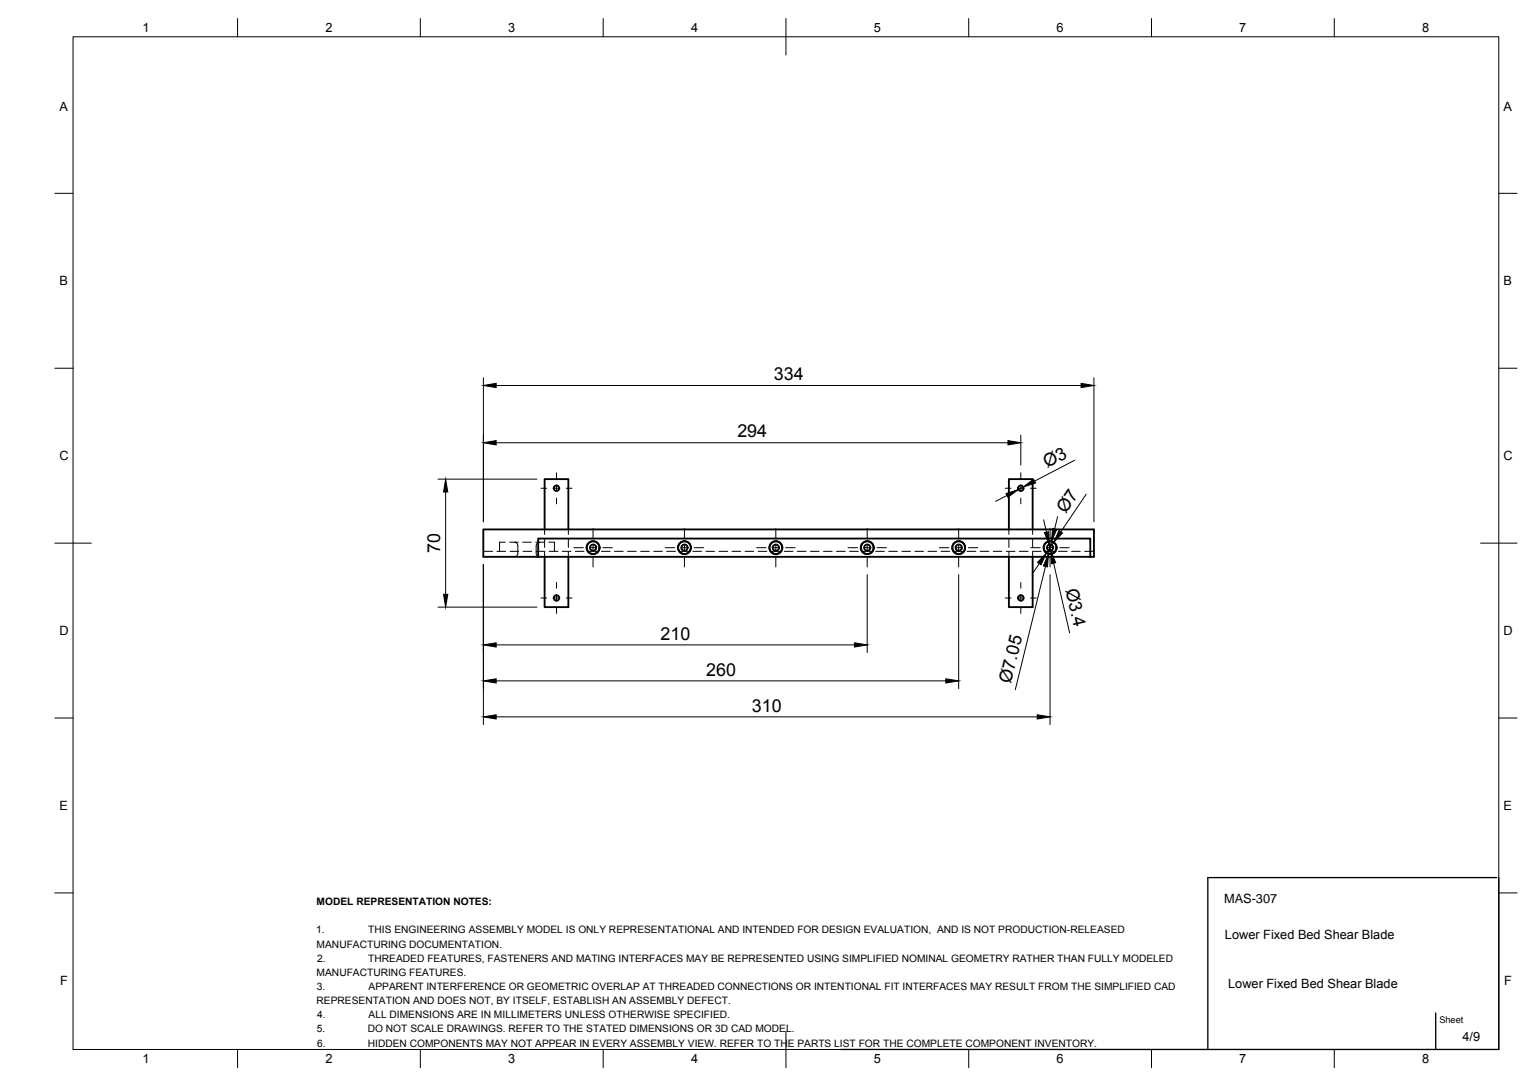
ISO-10303-21;
HEADER;
FILE_DESCRIPTION (('STEP AP214'),
    '1' );
FILE_NAME ('Lower Fixed Bed Shear Blade.step',
    '2026-10-06T07:34:29',
    ( '' ),
    ( '' ),
    'SwSTEP 2.0',
    'SolidWorks 2025',
    '' );
FILE_SCHEMA (( 'AUTOMOTIVE_DESIGN' ));
ENDSEC;

DATA;
#1=ORIENTED_EDGE ( 'NONE', *, *, #36, .T. ) ;
#8=ORIENTED_EDGE ( 'NONE', *, *, #9613, .T. ) ;
#9=EDGE_LOOP ( 'NONE', ( #498, #10940, #14960, #5861, #9835 ) ) ;
#14=LINE ( 'NONE', #12973, #6716 ) ;
#16=VECTOR ( 'NONE', #3003, 1000.000000000000000 ) ;
#17=EDGE_CURVE ( 'NONE', #5528, #10245, #15139, .T. ) ;
#23=DIRECTION ( 'NONE',  ( -0.000000000000000000, 1.156482317317871478E-16, -1.000000000000000000 ) ) ;
#27=ORIENTED_EDGE ( 'NONE', *, *, #13841, .F. ) ;
#29=VECTOR ( 'NONE', #1575, 1000.000000000000000 ) ;
#33=VECTOR ( 'NONE', #1804, 1000.000000000000000 ) ;
#36=EDGE_CURVE ( 'NONE', #15150, #10379, #8408, .T. ) ;
#43=DIRECTION ( 'NONE',  ( 0.000000000000000000, 0.000000000000000000, 1.000000000000000000 ) ) ;
#46=FACE_OUTER_BOUND ( 'NONE', #2849, .T. ) ;
#49=ORIENTED_EDGE ( 'NONE', *, *, #2623, .T. ) ;
#55=CARTESIAN_POINT ( 'NONE',  ( -76.50000000000001421, 19.53993994372674692, -17.50000000000002487 ) ) ;
#59=EDGE_CURVE ( 'NONE', #163, #6601, #13932, .T. ) ;
#61=VERTEX_POINT ( 'NONE', #1883 ) ;
#62=AXIS2_PLACEMENT_3D ( 'NONE', #15140, #11528, #6573 ) ;
#66=ORIENTED_EDGE ( 'NONE', *, *, #14903, .T. ) ;
#80=CIRCLE ( 'NONE', #13699, 3.525000000000000355 ) ;
#81=CARTESIAN_POINT ( 'NONE',  ( -110.0000000000000426, 59.53993994372674337, 10.00000000000000178 ) ) ;
#83=ADVANCED_FACE ( 'NONE', ( #687 ), #5531, .F. ) ;
#86=EDGE_LOOP ( 'NONE', ( #3348, #2604, #2165, #14498 ) ) ;
#93=ORIENTED_EDGE ( 'NONE', *, *, #2529, .F. ) ;
#94=AXIS2_PLACEMENT_3D ( 'NONE', #7418, #12210, #6221 ) ;
#111=ADVANCED_FACE ( 'NONE', ( #1394 ), #10899, .F. ) ;
#114=CARTESIAN_POINT ( 'NONE',  ( -35.99999999999995026, 62.13993994372673768, 18.50000000000140332 ) ) ;
#116=CARTESIAN_POINT ( 'NONE',  ( -108.0000000000000568, 64.53993994372673626, 20.00000000000000355 ) ) ;
#119=CARTESIAN_POINT ( 'NONE',  ( 114.0000000000000568, 64.53993994372673626, 11.50000000000034817 ) ) ;
#126=CARTESIAN_POINT ( 'NONE',  ( 185.1062858801516882, 25.86394065090268057, 18.00000000000000355 ) ) ;
#131=ORIENTED_EDGE ( 'NONE', *, *, #13724, .F. ) ;
#139=CARTESIAN_POINT ( 'NONE',  ( 164.0000000000000568, 64.53993994372673626, 16.70000000000000995 ) ) ;
#147=PLANE ( 'NONE',  #811 ) ;
#162=DIRECTION ( 'NONE',  ( 8.659560562354932858E-17, 0.7071067811865474617, -0.7071067811865474617 ) ) ;
#163=VERTEX_POINT ( 'NONE', #8301 ) ;
#167=ORIENTED_EDGE ( 'NONE', *, *, #13377, .T. ) ;
#178=CARTESIAN_POINT ( 'NONE',  ( -85.99999999999994316, 64.51493994372674479, 18.50000000000175149 ) ) ;
#181=CARTESIAN_POINT ( 'NONE',  ( 200.1062858801516597, 40.86394065090267702, 12.00000000000001066 ) ) ;
#186=DIRECTION ( 'NONE',  ( 0.000000000000000000, 0.000000000000000000, 1.000000000000000000 ) ) ;
#198=DIRECTION ( 'NONE',  ( 0.000000000000000000, 0.000000000000000000, 1.000000000000000000 ) ) ;
#210=EDGE_LOOP ( 'NONE', ( #10445, #12034, #11284, #6545 ) ) ;
#220=DIRECTION ( 'NONE',  ( -0.000000000000000000, 1.486905836551548832E-16, -1.000000000000000000 ) ) ;
#221=ORIENTED_EDGE ( 'NONE', *, *, #12224, .F. ) ;
#222=( GEOMETRIC_REPRESENTATION_CONTEXT ( 3 ) GLOBAL_UNCERTAINTY_ASSIGNED_CONTEXT ( ( #10529 ) ) GLOBAL_UNIT_ASSIGNED_CONTEXT ( ( #15547, #7222, #9271 ) ) REPRESENTATION_CONTEXT ( 'NONE', 'WORKASPACE' ) );
#232=DIRECTION ( 'NONE',  ( -0.000000000000000000, 1.000000000000000000, 1.156482317317871725E-16 ) ) ;
#233=AXIS2_PLACEMENT_3D ( 'NONE', #7331, #6137, #10957 ) ;
#236=LINE ( 'NONE', #6353, #3489 ) ;
#240=DIRECTION ( 'NONE',  ( 0.000000000000000000, -1.000000000000000000, 0.000000000000000000 ) ) ;
#244=EDGE_CURVE ( 'NONE', #1879, #4614, #5269, .T. ) ;
#250=ORIENTED_EDGE ( 'NONE', *, *, #12118, .T. ) ;
#252=CYLINDRICAL_SURFACE ( 'NONE', #13481, 1.700000000000007061 ) ;
#253=EDGE_CURVE ( 'NONE', #2275, #9404, #10915, .T. ) ;
#259=VERTEX_POINT ( 'NONE', #512 ) ;
#262=ADVANCED_FACE ( 'NONE', ( #11203, #355 ), #1639, .F. ) ;
#263=CARTESIAN_POINT ( 'NONE',  ( 14.00000000000004086, 64.53993994372673626, 15.00000000000104983 ) ) ;
#267=DIRECTION ( 'NONE',  ( 0.000000000000000000, -1.000000000000000000, -1.156482317317871478E-16 ) ) ;
#272=CARTESIAN_POINT ( 'NONE',  ( 14.00000000000004086, 62.13993994372673768, 15.00000000000104983 ) ) ;
#275=ORIENTED_EDGE ( 'NONE', *, *, #10508, .T. ) ;
#276=CARTESIAN_POINT ( 'NONE',  ( 215.1062858801516882, 55.86394065090267702, 13.00000000000000178 ) ) ;
#278=EDGE_CURVE ( 'NONE', #319, #8130, #1801, .T. ) ;
#280=DIRECTION ( 'NONE',  ( 0.000000000000000000, 0.000000000000000000, 1.000000000000000000 ) ) ;
#293=ORIENTED_EDGE ( 'NONE', *, *, #8057, .F. ) ;
#299=VERTEX_POINT ( 'NONE', #8683 ) ;
#300=DIRECTION ( 'NONE',  ( 0.000000000000000000, 1.000000000000000000, 0.000000000000000000 ) ) ;
#303=ORIENTED_EDGE ( 'NONE', *, *, #14000, .F. ) ;
#308=CARTESIAN_POINT ( 'NONE',  ( 177.5000000000000853, 17.53993994372673271, 52.49999999999997868 ) ) ;
#309=EDGE_LOOP ( 'NONE', ( #6645, #5526, #11534, #9026 ) ) ;
#312=COLOUR_RGB ( '', 0.08235294, 0.09019608, 0.10196078) ;
#315=ORIENTED_EDGE ( 'NONE', *, *, #1829, .T. ) ;
#319=VERTEX_POINT ( 'NONE', #10023 ) ;
#321=FACE_BOUND ( 'NONE', #9577, .T. ) ;
#324=FACE_OUTER_BOUND ( 'NONE', #11938, .T. ) ;
#327=DIRECTION ( 'NONE',  ( -0.000000000000000000, 1.000000000000000000, 0.000000000000000000 ) ) ;
#337=ORIENTED_EDGE ( 'NONE', *, *, #9909, .T. ) ;
#340=DIRECTION ( 'NONE',  ( -0.000000000000000000, 1.000000000000000000, -0.000000000000000000 ) ) ;
#346=EDGE_CURVE ( 'NONE', #13457, #11923, #1210, .T. ) ;
#348=DIRECTION ( 'NONE',  ( 0.000000000000000000, 0.000000000000000000, 1.000000000000000000 ) ) ;
#349=ORIENTED_EDGE ( 'NONE', *, *, #4874, .F. ) ;
#350=CARTESIAN_POINT ( 'NONE',  ( -70.00000000000000000, 19.53993994372674337, -12.49999999999999467 ) ) ;
#353=FACE_OUTER_BOUND ( 'NONE', #13566, .T. ) ;
#355=FACE_OUTER_BOUND ( 'NONE', #6775, .T. ) ;
#356=LINE ( 'NONE', #15042, #7156 ) ;
#357=CYLINDRICAL_SURFACE ( 'NONE', #6736, 1.700000000000001954 ) ;
#363=FACE_OUTER_BOUND ( 'NONE', #2322, .T. ) ;
#368=EDGE_LOOP ( 'NONE', ( #10873, #2288 ) ) ;
#370=ORIENTED_EDGE ( 'NONE', *, *, #1545, .F. ) ;
#382=EDGE_LOOP ( 'NONE', ( #11195, #13930, #5127, #3542 ) ) ;
#391=CARTESIAN_POINT ( 'NONE',  ( -85.99999999999994316, 62.13993994372673768, 13.30000000000175575 ) ) ;
#402=DIRECTION ( 'NONE',  ( -0.000000000000000000, 1.000000000000000000, -0.000000000000000000 ) ) ;
#404=FACE_BOUND ( 'NONE', #3437, .T. ) ;
#411=VERTEX_POINT ( 'NONE', #1368 ) ;
#413=CARTESIAN_POINT ( 'NONE',  ( -63.50000000000002842, 19.53993994372674337, 9.999999999999998224 ) ) ;
#422=EDGE_CURVE ( 'NONE', #8299, #5528, #13370, .T. ) ;
#428=ORIENTED_EDGE ( 'NONE', *, *, #9080, .F. ) ;
#432=CARTESIAN_POINT ( 'NONE',  ( -70.00000000000000000, 17.53993994372673271, 45.99999999999998579 ) ) ;
#435=VERTEX_POINT ( 'NONE', #5016 ) ;
#438=PRODUCT_DEFINITION_CONTEXT ( 'detailed design', #1607, 'design' ) ;
#449=CARTESIAN_POINT ( 'NONE',  ( 184.0000000000000568, 19.53993994372674337, -10.99999999999999822 ) ) ;
#464=AXIS2_PLACEMENT_3D ( 'NONE', #11793, #3266, #8332 ) ;
#467=EDGE_LOOP ( 'NONE', ( #5925, #93, #1050, #7042 ) ) ;
#469=LINE ( 'NONE', #13437, #12129 ) ;
#470=VERTEX_POINT ( 'NONE', #2334 ) ;
#473=CIRCLE ( 'NONE', #10842, 3.525000000000000355 ) ;
#487=ORIENTED_EDGE ( 'NONE', *, *, #5572, .T. ) ;
#490=ORIENTED_EDGE ( 'NONE', *, *, #10011, .F. ) ;
#497=CARTESIAN_POINT ( 'NONE',  ( -35.99999999999995026, 59.53993994372674337, 13.30000000000139870 ) ) ;
#498=ORIENTED_EDGE ( 'NONE', *, *, #7139, .T. ) ;
#499=FACE_OUTER_BOUND ( 'NONE', #8321, .T. ) ;
#504=ORIENTED_EDGE ( 'NONE', *, *, #12136, .F. ) ;
#512=CARTESIAN_POINT ( 'NONE',  ( 194.0000000000000568, 64.53993994372673626, 10.00000000000000178 ) ) ;
#521=AXIS2_PLACEMENT_3D ( 'NONE', #14117, #9393, #14192 ) ;
#527=ORIENTED_EDGE ( 'NONE', *, *, #1736, .T. ) ;
#546=ORIENTED_EDGE ( 'NONE', *, *, #11091, .T. ) ;
#560=DIRECTION ( 'NONE',  ( -0.000000000000000000, 1.000000000000000000, -0.000000000000000000 ) ) ;
#576=VECTOR ( 'NONE', #13961, 1000.000000000000000 ) ;
#591=VERTEX_POINT ( 'NONE', #3904 ) ;
#596=ADVANCED_FACE ( 'NONE', ( #3241, #7547, #404, #10066, #5321, #12343, #1529 ), #6365, .T. ) ;
#597=VECTOR ( 'NONE', #13500, 1000.000000000000000 ) ;
#598=CARTESIAN_POINT ( 'NONE',  ( 14.00000000000004086, 64.51493994372674479, 11.50000000000105160 ) ) ;
#605=FACE_OUTER_BOUND ( 'NONE', #8179, .T. ) ;
#608=CARTESIAN_POINT ( 'NONE',  ( 200.1062858801516597, 40.86394065090267702, 12.00000000000001066 ) ) ;
#613=CARTESIAN_POINT ( 'NONE',  ( 114.0000000000000568, 59.53993994372674337, 15.00000000000035172 ) ) ;
#614=CARTESIAN_POINT ( 'NONE',  ( 185.1062858801516882, 55.86394065090267702, 18.00000000000000355 ) ) ;
#625=EDGE_CURVE ( 'NONE', #15030, #13622, #4821, .T. ) ;
#627=VERTEX_POINT ( 'NONE', #2292 ) ;
#629=VECTOR ( 'NONE', #6503, 1000.000000000000114 ) ;
#634=VECTOR ( 'NONE', #8882, 1000.000000000000000 ) ;
#641=DIRECTION ( 'NONE',  ( 0.000000000000000000, 0.000000000000000000, 1.000000000000000000 ) ) ;
#644=DIRECTION ( 'NONE',  ( 0.000000000000000000, -1.000000000000000000, 0.000000000000000000 ) ) ;
#646=CARTESIAN_POINT ( 'NONE',  ( 114.0000000000000568, 59.53993994372674337, 13.30000000000035776 ) ) ;
#649=VERTEX_POINT ( 'NONE', #14359 ) ;
#659=EDGE_LOOP ( 'NONE', ( #14595, #131 ) ) ;
#662=FACE_OUTER_BOUND ( 'NONE', #4108, .T. ) ;
#665=DIRECTION ( 'NONE',  ( 0.000000000000000000, 0.000000000000000000, 1.000000000000000000 ) ) ;
#666=ORIENTED_EDGE ( 'NONE', *, *, #11149, .F. ) ;
#668=DIRECTION ( 'NONE',  ( 0.000000000000000000, 0.000000000000000000, -1.000000000000000000 ) ) ;
#669=DIRECTION ( 'NONE',  ( -0.000000000000000000, 1.000000000000000000, -0.000000000000000000 ) ) ;
#670=CARTESIAN_POINT ( 'NONE',  ( 164.0000000000000568, 62.13993994372673768, 15.00000000000000355 ) ) ;
#677=FACE_OUTER_BOUND ( 'NONE', #3082, .T. ) ;
#687=FACE_OUTER_BOUND ( 'NONE', #13168, .T. ) ;
#692=VECTOR ( 'NONE', #1638, 1000.000000000000000 ) ;
#694=ORIENTED_EDGE ( 'NONE', *, *, #8736, .F. ) ;
#701=VERTEX_POINT ( 'NONE', #11853 ) ;
#702=ORIENTED_EDGE ( 'NONE', *, *, #1006, .F. ) ;
#711=DIRECTION ( 'NONE',  ( 1.000000000000000000, 0.000000000000000000, 0.000000000000000000 ) ) ;
#712=DIRECTION ( 'NONE',  ( 1.000000000000000000, 0.000000000000000000, -0.000000000000000000 ) ) ;
#716=CARTESIAN_POINT ( 'NONE',  ( -70.00000000000000000, 17.53993994372673271, 47.49999999999997868 ) ) ;
#728=AXIS2_PLACEMENT_3D ( 'NONE', #4128, #8966, #3036 ) ;
#733=DIRECTION ( 'NONE',  ( 0.000000000000000000, 0.000000000000000000, 1.000000000000000000 ) ) ;
#737=AXIS2_PLACEMENT_3D ( 'NONE', #10217, #240, #15526 ) ;
#741=CYLINDRICAL_SURFACE ( 'NONE', #7444, 3.500000000000001332 ) ;
#747=EDGE_CURVE ( 'NONE', #6193, #15197, #6107, .T. ) ;
#755=CARTESIAN_POINT ( 'NONE',  ( 64.00000000000005684, 64.53993994372673626, 15.00000000000070166 ) ) ;
#759=CARTESIAN_POINT ( 'NONE',  ( 184.0000000000000568, 17.53993994372673271, 47.49999999999997868 ) ) ;
#774=CARTESIAN_POINT ( 'NONE',  ( 64.00000000000005684, 64.53993994372673626, 11.47500000000070131 ) ) ;
#778=ORIENTED_EDGE ( 'NONE', *, *, #7223, .T. ) ;
#782=ORIENTED_EDGE ( 'NONE', *, *, #1484, .F. ) ;
#786=DIRECTION ( 'NONE',  ( 0.000000000000000000, 0.000000000000000000, 1.000000000000000000 ) ) ;
#792=DIRECTION ( 'NONE',  ( 0.000000000000000000, -1.486905836551548832E-16, 1.000000000000000000 ) ) ;
#794=CARTESIAN_POINT ( 'NONE',  ( 14.00000000000004086, 59.53993994372674337, 15.00000000000104983 ) ) ;
#807=ORIENTED_EDGE ( 'NONE', *, *, #7985, .T. ) ;
#811=AXIS2_PLACEMENT_3D ( 'NONE', #8478, #2543, #7216 ) ;
#819=CARTESIAN_POINT ( 'NONE',  ( 200.1062858801516597, 40.86394065090267702, 12.00000000000001066 ) ) ;
#820=ADVANCED_FACE ( 'NONE', ( #7360 ), #12154, .F. ) ;
#821=AXIS2_PLACEMENT_3D ( 'NONE', #7186, #2427, #43 ) ;
#841=DIRECTION ( 'NONE',  ( 0.000000000000000000, -1.000000000000000000, 0.000000000000000000 ) ) ;
#842=CIRCLE ( 'NONE', #12444, 1.499999999999997780 ) ;
#843=DIRECTION ( 'NONE',  ( 0.000000000000000000, 0.000000000000000000, -1.000000000000000000 ) ) ;
#848=ORIENTED_EDGE ( 'NONE', *, *, #6781, .T. ) ;
#851=CIRCLE ( 'NONE', #6656, 1.499999999999997780 ) ;
#855=EDGE_CURVE ( 'NONE', #8929, #14758, #8389, .T. ) ;
#856=EDGE_CURVE ( 'NONE', #10437, #9262, #1951, .T. ) ;
#864=ORIENTED_EDGE ( 'NONE', *, *, #15101, .T. ) ;
#865=CYLINDRICAL_SURFACE ( 'NONE', #11752, 1.699999999999994849 ) ;
#868=VERTEX_POINT ( 'NONE', #5283 ) ;
#871=CARTESIAN_POINT ( 'NONE',  ( 200.1062858801516597, 40.86394065090267702, 16.00000000000001421 ) ) ;
#889=EDGE_CURVE ( 'NONE', #9525, #12618, #11656, .T. ) ;
#891=DIRECTION ( 'NONE',  ( 0.000000000000000000, 1.000000000000000000, 1.156482317317871725E-16 ) ) ;
#899=VERTEX_POINT ( 'NONE', #14266 ) ;
#903=DIRECTION ( 'NONE',  ( 0.000000000000000000, 0.000000000000000000, 1.000000000000000000 ) ) ;
#910=CARTESIAN_POINT ( 'NONE',  ( 64.00000000000005684, 62.13993994372673768, 15.00000000000070166 ) ) ;
#912=CARTESIAN_POINT ( 'NONE',  ( -35.99999999999995026, 62.13993994372673768, 15.00000000000139977 ) ) ;
#917=EDGE_CURVE ( 'NONE', #11949, #9422, #12929, .T. ) ;
#922=CARTESIAN_POINT ( 'NONE',  ( -35.99999999999995026, 59.53993994372674337, 13.30000000000139870 ) ) ;
#925=DIRECTION ( 'NONE',  ( -1.000000000000000000, -0.000000000000000000, -0.000000000000000000 ) ) ;
#926=ORIENTED_EDGE ( 'NONE', *, *, #13201, .T. ) ;
#929=CIRCLE ( 'NONE', #7000, 2.000000000000000000 ) ;
#931=DIRECTION ( 'NONE',  ( 1.000000000000000000, 0.000000000000000000, 0.000000000000000000 ) ) ;
#936=VECTOR ( 'NONE', #12404, 1000.000000000000000 ) ;
#941=CARTESIAN_POINT ( 'NONE',  ( -108.0000000000000568, 64.53993994372673626, 20.00000000000000355 ) ) ;
#953=CIRCLE ( 'NONE', #1966, 3.500000000000003109 ) ;
#954=DIRECTION ( 'NONE',  ( -0.000000000000000000, 1.000000000000000000, 1.156482317317871725E-16 ) ) ;
#957=CARTESIAN_POINT ( 'NONE',  ( 0.000000000000000000, 19.53993994372674337, 2.905405074819403421E-15 ) ) ;
#958=ORIENTED_EDGE ( 'NONE', *, *, #14050, .F. ) ;
#959=CARTESIAN_POINT ( 'NONE',  ( 64.00000000000005684, 64.53993994372673626, 16.70000000000069207 ) ) ;
#960=AXIS2_PLACEMENT_3D ( 'NONE', #2650, #2411, #6129 ) ;
#968=CARTESIAN_POINT ( 'NONE',  ( 194.0000000000000568, 26.39124795404934076, 0.000000000000000000 ) ) ;
#973=VERTEX_POINT ( 'NONE', #9469 ) ;
#979=VECTOR ( 'NONE', #3430, 1000.000000000000000 ) ;
#984=ADVANCED_FACE ( 'NONE', ( #6951, #7191 ), #3540, .T. ) ;
#988=FACE_BOUND ( 'NONE', #7044, .T. ) ;
#990=LINE ( 'NONE', #10329, #3876 ) ;
#991=LINE ( 'NONE', #2500, #12258 ) ;
#993=VECTOR ( 'NONE', #10687, 1000.000000000000000 ) ;
#998=EDGE_CURVE ( 'NONE', #9262, #11923, #11758, .T. ) ;
#999=PLANE ( 'NONE',  #14722 ) ;
#1006=EDGE_CURVE ( 'NONE', #4775, #10379, #5752, .T. ) ;
#1009=ORIENTED_EDGE ( 'NONE', *, *, #8860, .T. ) ;
#1014=CARTESIAN_POINT ( 'NONE',  ( 190.5000000000000568, 17.53993994372674692, -17.50000000000002487 ) ) ;
#1017=CIRCLE ( 'NONE', #6335, 3.500000000000003109 ) ;
#1019=AXIS2_PLACEMENT_3D ( 'NONE', #10169, #11272, #4150 ) ;
#1023=ORIENTED_EDGE ( 'NONE', *, *, #4835, .T. ) ;
#1024=DIRECTION ( 'NONE',  ( -0.000000000000000000, 1.000000000000000000, -0.000000000000000000 ) ) ;
#1026=EDGE_CURVE ( 'NONE', #8395, #4264, #11155, .T. ) ;
#1045=ORIENTED_EDGE ( 'NONE', *, *, #6433, .F. ) ;
#1050=ORIENTED_EDGE ( 'NONE', *, *, #11057, .F. ) ;
#1057=VECTOR ( 'NONE', #10570, 1000.000000000000000 ) ;
#1065=LINE ( 'NONE', #10870, #11730 ) ;
#1068=DIRECTION ( 'NONE',  ( 0.000000000000000000, 0.000000000000000000, 1.000000000000000000 ) ) ;
#1069=AXIS2_PLACEMENT_3D ( 'NONE', #6183, #9807, #13259 ) ;
#1070=LINE ( 'NONE', #10710, #2815 ) ;
#1075=CYLINDRICAL_SURFACE ( 'NONE', #12938, 1.699999999999991518 ) ;
#1076=DIRECTION ( 'NONE',  ( 0.000000000000000000, 0.000000000000000000, -1.000000000000000000 ) ) ;
#1083=LINE ( 'NONE', #6073, #2781 ) ;
#1087=EDGE_CURVE ( 'NONE', #6095, #12779, #3924, .T. ) ;
#1091=AXIS2_PLACEMENT_3D ( 'NONE', #5904, #14335, #10721 ) ;
#1093=FACE_OUTER_BOUND ( 'NONE', #8112, .T. ) ;
#1095=VECTOR ( 'NONE', #6395, 1000.000000000000000 ) ;
#1104=AXIS2_PLACEMENT_3D ( 'NONE', #6378, #3194, #15329 ) ;
#1108=LINE ( 'NONE', #1260, #15580 ) ;
#1110=ORIENTED_EDGE ( 'NONE', *, *, #1281, .F. ) ;
#1114=EDGE_CURVE ( 'NONE', #6055, #3552, #2548, .T. ) ;
#1122=AXIS2_PLACEMENT_3D ( 'NONE', #11812, #7243, #8431 ) ;
#1133=VECTOR ( 'NONE', #9502, 1000.000000000000000 ) ;
#1134=ORIENTED_EDGE ( 'NONE', *, *, #3215, .F. ) ;
#1147=ORIENTED_EDGE ( 'NONE', *, *, #3050, .T. ) ;
#1148=ORIENTED_EDGE ( 'NONE', *, *, #17, .F. ) ;
#1150=FACE_BOUND ( 'NONE', #2621, .T. ) ;
#1151=ADVANCED_FACE ( 'NONE', ( #13538 ), #13394, .F. ) ;
#1161=VERTEX_POINT ( 'NONE', #5190 ) ;
#1164=DIRECTION ( 'NONE',  ( -0.000000000000000000, 1.000000000000000000, -0.000000000000000000 ) ) ;
#1166=SURFACE_STYLE_USAGE ( .BOTH. , #11997 ) ;
#1169=DIRECTION ( 'NONE',  ( -0.000000000000000000, 1.000000000000000000, -0.000000000000000000 ) ) ;
#1182=EDGE_LOOP ( 'NONE', ( #11077, #12409, #5539, #8357 ) ) ;
#1183=CARTESIAN_POINT ( 'NONE',  ( 190.5000000000000853, 17.53993994372673271, 52.49999999999997868 ) ) ;
#1209=ORIENTED_EDGE ( 'NONE', *, *, #9778, .T. ) ;
#1210=LINE ( 'NONE', #12263, #6859 ) ;
#1219=ORIENTED_EDGE ( 'NONE', *, *, #14249, .T. ) ;
#1220=ADVANCED_FACE ( 'NONE', ( #10165 ), #15113, .F. ) ;
#1239=CIRCLE ( 'NONE', #6307, 3.500000000000001332 ) ;
#1242=AXIS2_PLACEMENT_3D ( 'NONE', #12493, #11401, #7940 ) ;
#1245=DIRECTION ( 'NONE',  ( -0.000000000000000000, 1.000000000000000000, 1.156482317317871725E-16 ) ) ;
#1246=PLANE ( 'NONE',  #7999 ) ;
#1248=CARTESIAN_POINT ( 'NONE',  ( 14.00000000000004086, 64.53993994372673626, 15.00000000000104983 ) ) ;
#1251=EDGE_CURVE ( 'NONE', #9250, #11935, #13867, .T. ) ;
#1253=AXIS2_PLACEMENT_3D ( 'NONE', #3458, #10965, #5829 ) ;
#1260=CARTESIAN_POINT ( 'NONE',  ( -35.99999999999995026, 64.53993994372673626, 11.50000000000139622 ) ) ;
#1266=AXIS2_PLACEMENT_3D ( 'NONE', #9362, #6996, #2090 ) ;
#1277=CARTESIAN_POINT ( 'NONE',  ( -70.00000000000000000, 19.53993994372674337, -13.99999999999999289 ) ) ;
#1281=EDGE_CURVE ( 'NONE', #11184, #10896, #473, .T. ) ;
#1287=AXIS2_PLACEMENT_3D ( 'NONE', #5372, #9089, #4100 ) ;
#1300=CARTESIAN_POINT ( 'NONE',  ( 114.0000000000000568, 64.53993994372673626, 11.47500000000035136 ) ) ;
#1302=ORIENTED_EDGE ( 'NONE', *, *, #9805, .T. ) ;
#1307=CARTESIAN_POINT ( 'NONE',  ( -110.0000000000000426, 59.53993994372674337, 10.00000000000000178 ) ) ;
#1313=EDGE_CURVE ( 'NONE', #9986, #11722, #5261, .T. ) ;
#1317=DIRECTION ( 'NONE',  ( -0.000000000000000000, 1.000000000000000000, -0.000000000000000000 ) ) ;
#1318=DIRECTION ( 'NONE',  ( 1.000000000000000000, 0.000000000000000000, 0.000000000000000000 ) ) ;
#1319=EDGE_LOOP ( 'NONE', ( #14221, #12598, #7572, #3944 ) ) ;
#1322=CARTESIAN_POINT ( 'NONE',  ( 200.1062858801516597, 40.86394065090267702, 16.00000000000001421 ) ) ;
#1324=CARTESIAN_POINT ( 'NONE',  ( -110.0000000000000426, 19.53993994372674337, 9.999999999999998224 ) ) ;
#1326=DIRECTION ( 'NONE',  ( 0.000000000000000000, 0.000000000000000000, 1.000000000000000000 ) ) ;
#1327=CARTESIAN_POINT ( 'NONE',  ( 164.0000000000000568, 64.53993994372673626, 11.50000000000000000 ) ) ;
#1338=CARTESIAN_POINT ( 'NONE',  ( 14.00000000000004086, 62.13993994372673768, 13.30000000000105054 ) ) ;
#1339=VECTOR ( 'NONE', #10249, 1000.000000000000000 ) ;
#1340=EDGE_LOOP ( 'NONE', ( #7669, #13345 ) ) ;
#1359=AXIS2_PLACEMENT_3D ( 'NONE', #7035, #4487, #13008 ) ;
#1364=ADVANCED_FACE ( 'NONE', ( #11665 ), #11815, .F. ) ;
#1368=CARTESIAN_POINT ( 'NONE',  ( -70.00000000000000000, 17.53993994372673271, 48.99999999999997158 ) ) ;
#1372=ORIENTED_EDGE ( 'NONE', *, *, #9556, .F. ) ;
#1377=CONICAL_SURFACE ( 'NONE', #8712, 3.525000000000002132, 0.7853981633974482790 ) ;
#1389=AXIS2_PLACEMENT_3D ( 'NONE', #6841, #13934, #11495 ) ;
#1391=EDGE_LOOP ( 'NONE', ( #428, #6702, #6658, #10982 ) ) ;
#1394=FACE_OUTER_BOUND ( 'NONE', #1997, .T. ) ;
#1395=CARTESIAN_POINT ( 'NONE',  ( -35.99999999999995026, 64.53993994372673626, 11.47500000000139941 ) ) ;
#1398=EDGE_CURVE ( 'NONE', #11305, #13329, #8573, .T. ) ;
#1400=DIRECTION ( 'NONE',  ( 1.000000000000000000, 0.000000000000000000, -0.000000000000000000 ) ) ;
#1405=CARTESIAN_POINT ( 'NONE',  ( 200.1062858801516597, 47.86394065090266992, 12.00000000000001066 ) ) ;
#1424=ORIENTED_EDGE ( 'NONE', *, *, #9453, .T. ) ;
#1425=CYLINDRICAL_SURFACE ( 'NONE', #3896, 3.500000000000004885 ) ;
#1427=DIRECTION ( 'NONE',  ( 0.000000000000000000, 0.000000000000000000, -1.000000000000000000 ) ) ;
#1428=ADVANCED_FACE ( 'NONE', ( #5661 ), #8831, .F. ) ;
#1429=DIRECTION ( 'NONE',  ( -0.000000000000000000, 1.000000000000000000, 1.156482317317871725E-16 ) ) ;
#1430=ORIENTED_EDGE ( 'NONE', *, *, #13657, .T. ) ;
#1434=VERTEX_POINT ( 'NONE', #11741 ) ;
#1443=CIRCLE ( 'NONE', #3225, 1.699999999999991518 ) ;
#1445=EDGE_CURVE ( 'NONE', #4264, #5504, #10547, .T. ) ;
#1457=CARTESIAN_POINT ( 'NONE',  ( 184.0000000000000568, 17.53993994372673271, 47.49999999999997868 ) ) ;
#1461=CARTESIAN_POINT ( 'NONE',  ( -85.99999999999994316, 64.53993994372673626, 15.00000000000174794 ) ) ;
#1466=VECTOR ( 'NONE', #14942, 1000.000000000000000 ) ;
#1467=VERTEX_POINT ( 'NONE', #8361 ) ;
#1470=CARTESIAN_POINT ( 'NONE',  ( 14.00000000000004086, 56.53993994372675047, 15.00000000000104983 ) ) ;
#1473=DIRECTION ( 'NONE',  ( 0.000000000000000000, -0.000000000000000000, -1.000000000000000000 ) ) ;
#1484=EDGE_CURVE ( 'NONE', #5113, #9730, #1239, .T. ) ;
#1495=CARTESIAN_POINT ( 'NONE',  ( 64.00000000000005684, 62.13993994372673768, 18.50000000000070344 ) ) ;
#1496=CARTESIAN_POINT ( 'NONE',  ( 114.0000000000000568, 62.13993994372673768, 18.50000000000035527 ) ) ;
#1500=VECTOR ( 'NONE', #644, 1000.000000000000000 ) ;
#1512=DIRECTION ( 'NONE',  ( 0.000000000000000000, 0.000000000000000000, -1.000000000000000000 ) ) ;
#1514=ORIENTED_EDGE ( 'NONE', *, *, #14251, .T. ) ;
#1516=LINE ( 'NONE', #14770, #5762 ) ;
#1521=CARTESIAN_POINT ( 'NONE',  ( 14.00000000000004086, 64.53993994372673626, 15.00000000000104983 ) ) ;
#1524=CIRCLE ( 'NONE', #7851, 3.500000000000004885 ) ;
#1525=AXIS2_PLACEMENT_3D ( 'NONE', #12830, #11509, #665 ) ;
#1526=FACE_BOUND ( 'NONE', #14844, .T. ) ;
#1528=ORIENTED_EDGE ( 'NONE', *, *, #856, .T. ) ;
#1529=FACE_OUTER_BOUND ( 'NONE', #13428, .T. ) ;
#1541=ADVANCED_FACE ( 'NONE', ( #1150, #3524, #988, #13143, #2345, #5740, #10554 ), #10797, .T. ) ;
#1545=EDGE_CURVE ( 'NONE', #10399, #9297, #13597, .T. ) ;
#1560=LINE ( 'NONE', #8837, #1095 ) ;
#1569=DIRECTION ( 'NONE',  ( 0.000000000000000000, 0.000000000000000000, -1.000000000000000000 ) ) ;
#1570=ORIENTED_EDGE ( 'NONE', *, *, #1313, .F. ) ;
#1573=CARTESIAN_POINT ( 'NONE',  ( -108.0000000000000568, 59.53993994372674337, 10.00000000000000178 ) ) ;
#1574=VECTOR ( 'NONE', #11068, 1000.000000000000000 ) ;
#1575=DIRECTION ( 'NONE',  ( 1.000000000000000000, 0.000000000000000000, 0.000000000000000000 ) ) ;
#1579=ADVANCED_FACE ( 'NONE', ( #10057, #2953 ), #12645, .F. ) ;
#1580=CARTESIAN_POINT ( 'NONE',  ( 14.00000000000004086, 59.53993994372674337, 15.00000000000104983 ) ) ;
#1585=AXIS2_PLACEMENT_3D ( 'NONE', #4159, #11516, #10332 ) ;
#1586=DIRECTION ( 'NONE',  ( 0.000000000000000000, 0.000000000000000000, 1.000000000000000000 ) ) ;
#1599=AXIS2_PLACEMENT_3D ( 'NONE', #10491, #6867, #11596 ) ;
#1601=LINE ( 'NONE', #4047, #634 ) ;
#1607=APPLICATION_CONTEXT ( 'automotive_design' ) ;
#1616=ORIENTED_EDGE ( 'NONE', *, *, #15191, .T. ) ;
#1622=DIRECTION ( 'NONE',  ( -0.000000000000000000, 1.000000000000000000, -0.000000000000000000 ) ) ;
#1627=ORIENTED_EDGE ( 'NONE', *, *, #9905, .T. ) ;
#1628=CYLINDRICAL_SURFACE ( 'NONE', #6182, 1.700000000000007061 ) ;
#1635=ORIENTED_EDGE ( 'NONE', *, *, #3279, .T. ) ;
#1636=ORIENTED_EDGE ( 'NONE', *, *, #59, .T. ) ;
#1638=DIRECTION ( 'NONE',  ( 1.000000000000000000, 0.000000000000000000, 0.000000000000000000 ) ) ;
#1639=PLANE ( 'NONE',  #7391 ) ;
#1640=DIRECTION ( 'NONE',  ( 0.000000000000000000, 0.000000000000000000, 1.000000000000000000 ) ) ;
#1646=DIRECTION ( 'NONE',  ( 1.000000000000000000, -4.585547486636276518E-32, 3.965082230804130220E-16 ) ) ;
#1647=DIRECTION ( 'NONE',  ( -0.000000000000000000, 1.000000000000000000, -0.000000000000000000 ) ) ;
#1654=LINE ( 'NONE', #15057, #16 ) ;
#1659=VECTOR ( 'NONE', #10535, 1000.000000000000000 ) ;
#1664=CARTESIAN_POINT ( 'NONE',  ( 200.1062858801516597, 40.86394065090267702, 12.00000000000001066 ) ) ;
#1668=CARTESIAN_POINT ( 'NONE',  ( -110.0000000000000426, 26.39124795404934076, 0.000000000000000000 ) ) ;
#1683=DIRECTION ( 'NONE',  ( -0.000000000000000000, 1.000000000000000000, -0.000000000000000000 ) ) ;
#1684=ORIENTED_EDGE ( 'NONE', *, *, #278, .T. ) ;
#1700=VERTEX_POINT ( 'NONE', #14929 ) ;
#1703=ADVANCED_FACE ( 'NONE', ( #7698 ), #12487, .F. ) ;
#1710=EDGE_LOOP ( 'NONE', ( #1528, #10910, #10729, #12950 ) ) ;
#1714=DIRECTION ( 'NONE',  ( -0.000000000000000000, 1.000000000000000000, -0.000000000000000000 ) ) ;
#1732=DIRECTION ( 'NONE',  ( 0.000000000000000000, 0.000000000000000000, -1.000000000000000000 ) ) ;
#1734=CIRCLE ( 'NONE', #10562, 6.999999999999978684 ) ;
#1736=EDGE_CURVE ( 'NONE', #10382, #2412, #10093, .T. ) ;
#1738=EDGE_LOOP ( 'NONE', ( #1372, #10188, #13821, #11406 ) ) ;
#1743=EDGE_LOOP ( 'NONE', ( #13760, #10131, #807, #7421 ) ) ;
#1745=AXIS2_PLACEMENT_3D ( 'NONE', #5566, #11325, #7871 ) ;
#1750=CARTESIAN_POINT ( 'NONE',  ( -35.99999999999995026, 56.53993994372675047, 15.00000000000139977 ) ) ;
#1751=ORIENTED_EDGE ( 'NONE', *, *, #2238, .F. ) ;
#1755=AXIS2_PLACEMENT_3D ( 'NONE', #14090, #6934, #903 ) ;
#1760=VECTOR ( 'NONE', #5317, 1000.000000000000000 ) ;
#1761=PLANE ( 'NONE',  #2765 ) ;
#1768=CARTESIAN_POINT ( 'NONE',  ( 184.0000000000000568, 17.53993994372673981, -10.99999999999999822 ) ) ;
#1773=CARTESIAN_POINT ( 'NONE',  ( 164.0000000000000568, 64.51493994372674479, 11.50000000000000000 ) ) ;
#1777=CIRCLE ( 'NONE', #5065, 1.499999999999997780 ) ;
#1796=EDGE_CURVE ( 'NONE', #4264, #8395, #6075, .T. ) ;
#1801=CIRCLE ( 'NONE', #15143, 3.500000000000003109 ) ;
#1804=DIRECTION ( 'NONE',  ( 0.000000000000000000, 1.000000000000000000, 0.000000000000000000 ) ) ;
#1805=ORIENTED_EDGE ( 'NONE', *, *, #4140, .T. ) ;
#1817=ORIENTED_EDGE ( 'NONE', *, *, #7244, .F. ) ;
#1829=EDGE_CURVE ( 'NONE', #4912, #5662, #3336, .T. ) ;
#1832=DIRECTION ( 'NONE',  ( 0.000000000000000000, -0.000000000000000000, -1.000000000000000000 ) ) ;
#1833=CARTESIAN_POINT ( 'NONE',  ( -110.0000000000000426, 22.53993994372673981, 24.99999999999999645 ) ) ;
#1837=CYLINDRICAL_SURFACE ( 'NONE', #3271, 1.699999999999996625 ) ;
#1879=VERTEX_POINT ( 'NONE', #11634 ) ;
#1880=EDGE_CURVE ( 'NONE', #10586, #12024, #6900, .T. ) ;
#1883=CARTESIAN_POINT ( 'NONE',  ( -108.0000000000000568, 64.53993994372673626, 10.00000000000000178 ) ) ;
#1902=ORIENTED_EDGE ( 'NONE', *, *, #4463, .T. ) ;
#1905=ORIENTED_EDGE ( 'NONE', *, *, #10039, .T. ) ;
#1907=LINE ( 'NONE', #2222, #12357 ) ;
#1908=EDGE_CURVE ( 'NONE', #8130, #2947, #1907, .T. ) ;
#1909=CARTESIAN_POINT ( 'NONE',  ( 64.00000000000005684, 64.51493994372674479, 18.50000000000070344 ) ) ;
#1910=DIRECTION ( 'NONE',  ( 0.000000000000000000, 0.000000000000000000, 1.000000000000000000 ) ) ;
#1911=CARTESIAN_POINT ( 'NONE',  ( 184.0000000000000568, 17.53993994372673271, 47.49999999999997868 ) ) ;
#1924=DIRECTION ( 'NONE',  ( -0.000000000000000000, 1.000000000000000000, -0.000000000000000000 ) ) ;
#1928=CARTESIAN_POINT ( 'NONE',  ( 0.000000000000000000, 19.53993994372674337, 2.905405074819403421E-15 ) ) ;
#1930=EDGE_LOOP ( 'NONE', ( #13294, #7913, #5232, #9705, #8762, #1514 ) ) ;
#1933=CARTESIAN_POINT ( 'NONE',  ( 14.00000000000004086, 64.53993994372673626, 15.00000000000104983 ) ) ;
#1938=EDGE_LOOP ( 'NONE', ( #2435, #14717, #9875, #7857 ) ) ;
#1939=DIRECTION ( 'NONE',  ( 3.965082230804130220E-16, -1.486905836551548832E-16, 1.000000000000000000 ) ) ;
#1940=CARTESIAN_POINT ( 'NONE',  ( 14.00000000000004086, 64.53993994372673626, 11.50000000000105160 ) ) ;
#1941=DIRECTION ( 'NONE',  ( 0.000000000000000000, 0.000000000000000000, 1.000000000000000000 ) ) ;
#1946=FACE_OUTER_BOUND ( 'NONE', #9084, .T. ) ;
#1951=LINE ( 'NONE', #12531, #33 ) ;
#1952=EDGE_LOOP ( 'NONE', ( #167, #14824, #4080, #14115, #2555, #13580, #2871, #3149 ) ) ;
#1953=CONICAL_SURFACE ( 'NONE', #14548, 3.524999999999998579, 0.7853981633974482790 ) ;
#1959=CYLINDRICAL_SURFACE ( 'NONE', #13197, 1.699999999999993072 ) ;
#1966=AXIS2_PLACEMENT_3D ( 'NONE', #11193, #14569, #3770 ) ;
#1985=DIRECTION ( 'NONE',  ( -1.000000000000000000, -0.000000000000000000, -0.000000000000000000 ) ) ;
#1988=EDGE_CURVE ( 'NONE', #10586, #5590, #12098, .T. ) ;
#1993=ORIENTED_EDGE ( 'NONE', *, *, #15375, .F. ) ;
#1994=DIRECTION ( 'NONE',  ( 0.000000000000000000, 0.000000000000000000, 1.000000000000000000 ) ) ;
#1997=EDGE_LOOP ( 'NONE', ( #2216, #13119, #7159, #10044 ) ) ;
#2004=CARTESIAN_POINT ( 'NONE',  ( -70.00000000000000000, 17.53993994372673981, -10.99999999999999822 ) ) ;
#2024=CIRCLE ( 'NONE', #1525, 1.700000000000001954 ) ;
#2026=VECTOR ( 'NONE', #12664, 1000.000000000000000 ) ;
#2031=PLANE ( 'NONE',  #1599 ) ;
#2037=ORIENTED_EDGE ( 'NONE', *, *, #5828, .F. ) ;
#2044=DIRECTION ( 'NONE',  ( -0.000000000000000000, 1.000000000000000000, -0.000000000000000000 ) ) ;
#2047=EDGE_CURVE ( 'NONE', #11935, #4694, #4914, .T. ) ;
#2051=EDGE_CURVE ( 'NONE', #5037, #299, #9803, .T. ) ;
#2054=AXIS2_PLACEMENT_3D ( 'NONE', #12743, #5498, #15107 ) ;
#2055=DIRECTION ( 'NONE',  ( -0.000000000000000000, 1.000000000000000000, -0.000000000000000000 ) ) ;
#2058=ORIENTED_EDGE ( 'NONE', *, *, #6781, .F. ) ;
#2061=FACE_BOUND ( 'NONE', #14693, .T. ) ;
#2073=CARTESIAN_POINT ( 'NONE',  ( 64.00000000000005684, 64.53993994372673626, 15.00000000000070166 ) ) ;
#2075=CARTESIAN_POINT ( 'NONE',  ( 200.1062858801516597, 45.86394065090266992, 12.00000000000001066 ) ) ;
#2084=EDGE_CURVE ( 'NONE', #15428, #8632, #4294, .T. ) ;
#2086=CARTESIAN_POINT ( 'NONE',  ( -70.00000000000000000, 19.53993994372674337, -10.99999999999999822 ) ) ;
#2090=DIRECTION ( 'NONE',  ( 0.000000000000000000, 0.000000000000000000, -1.000000000000000000 ) ) ;
#2093=DIRECTION ( 'NONE',  ( -0.000000000000000000, 1.000000000000000000, 1.486905836551548832E-16 ) ) ;
#2094=DIRECTION ( 'NONE',  ( 0.000000000000000000, 0.000000000000000000, 1.000000000000000000 ) ) ;
#2101=DIRECTION ( 'NONE',  ( -0.000000000000000000, 1.000000000000000000, -0.000000000000000000 ) ) ;
#2106=CARTESIAN_POINT ( 'NONE',  ( 114.0000000000000568, 59.53993994372674337, 15.00000000000035172 ) ) ;
#2107=DIRECTION ( 'NONE',  ( 0.000000000000000000, 0.000000000000000000, 1.000000000000000000 ) ) ;
#2113=AXIS2_PLACEMENT_3D ( 'NONE', #6139, #5978, #10959 ) ;
#2117=DIRECTION ( 'NONE',  ( 0.000000000000000000, 1.000000000000000000, 0.000000000000000000 ) ) ;
#2119=ORIENTED_EDGE ( 'NONE', *, *, #10977, .T. ) ;
#2127=ORIENTED_EDGE ( 'NONE', *, *, #8471, .T. ) ;
#2133=ORIENTED_EDGE ( 'NONE', *, *, #8002, .F. ) ;
#2134=FACE_OUTER_BOUND ( 'NONE', #14405, .T. ) ;
#2137=VERTEX_POINT ( 'NONE', #12394 ) ;
#2139=DIRECTION ( 'NONE',  ( 0.000000000000000000, 0.000000000000000000, -1.000000000000000000 ) ) ;
#2145=CYLINDRICAL_SURFACE ( 'NONE', #8084, 1.499999999999994449 ) ;
#2149=FILL_AREA_STYLE_COLOUR ( '', #12345 ) ;
#2158=EDGE_LOOP ( 'NONE', ( #9288, #2472 ) ) ;
#2160=CARTESIAN_POINT ( 'NONE',  ( -110.0000000000000426, 19.53993994372674337, 9.999999999999998224 ) ) ;
#2163=EDGE_CURVE ( 'NONE', #7275, #15150, #13731, .T. ) ;
#2165=ORIENTED_EDGE ( 'NONE', *, *, #5654, .T. ) ;
#2171=VERTEX_POINT ( 'NONE', #12626 ) ;
#2176=EDGE_CURVE ( 'NONE', #4254, #11465, #1524, .T. ) ;
#2198=( NAMED_UNIT ( * ) SI_UNIT ( $, .STERADIAN. ) SOLID_ANGLE_UNIT ( ) );
#2203=CARTESIAN_POINT ( 'NONE',  ( 64.00000000000005684, 64.51493994372674479, 15.00000000000070166 ) ) ;
#2204=CARTESIAN_POINT ( 'NONE',  ( -85.99999999999994316, 64.53993994372673626, 15.00000000000174794 ) ) ;
#2205=CARTESIAN_POINT ( 'NONE',  ( 164.0000000000000568, 56.53993994372675047, 13.29999999999999538 ) ) ;
#2210=VERTEX_POINT ( 'NONE', #1496 ) ;
#2216=ORIENTED_EDGE ( 'NONE', *, *, #4024, .T. ) ;
#2217=VERTEX_POINT ( 'NONE', #8702 ) ;
#2222=CARTESIAN_POINT ( 'NONE',  ( 164.0000000000000568, 64.53993994372673626, 18.50000000000000711 ) ) ;
#2232=ADVANCED_FACE ( 'NONE', ( #9967 ), #11147, .F. ) ;
#2238=EDGE_CURVE ( 'NONE', #6121, #2947, #1017, .T. ) ;
#2244=VECTOR ( 'NONE', #232, 1000.000000000000000 ) ;
#2255=AXIS2_PLACEMENT_3D ( 'NONE', #7461, #12257, #14467 ) ;
#2260=LINE ( 'NONE', #7330, #4538 ) ;
#2262=EDGE_CURVE ( 'NONE', #8929, #9928, #5687, .T. ) ;
#2264=CARTESIAN_POINT ( 'NONE',  ( 193.1062858801516882, 40.86394065090267702, 18.00000000000001066 ) ) ;
#2265=VECTOR ( 'NONE', #3204, 1000.000000000000000 ) ;
#2267=AXIS2_PLACEMENT_3D ( 'NONE', #12719, #10820, #8529 ) ;
#2273=AXIS2_PLACEMENT_3D ( 'NONE', #7860, #4271, #11240 ) ;
#2275=VERTEX_POINT ( 'NONE', #2205 ) ;
#2288=ORIENTED_EDGE ( 'NONE', *, *, #7223, .F. ) ;
#2289=AXIS2_PLACEMENT_3D ( 'NONE', #6935, #12674, #9375 ) ;
#2292=CARTESIAN_POINT ( 'NONE',  ( 14.00000000000004086, 62.13993994372673768, 16.70000000000105089 ) ) ;
#2294=CARTESIAN_POINT ( 'NONE',  ( -35.99999999999995026, 56.53993994372675047, 15.00000000000139977 ) ) ;
#2296=VERTEX_POINT ( 'NONE', #8155 ) ;
#2299=DIRECTION ( 'NONE',  ( 0.000000000000000000, 1.156482317317871478E-16, -1.000000000000000000 ) ) ;
#2306=ORIENTED_EDGE ( 'NONE', *, *, #14175, .T. ) ;
#2322=EDGE_LOOP ( 'NONE', ( #9063, #9365, #1627, #14599, #3492, #10575 ) ) ;
#2325=DIRECTION ( 'NONE',  ( -0.000000000000000000, -0.000000000000000000, -1.000000000000000000 ) ) ;
#2334=CARTESIAN_POINT ( 'NONE',  ( 205.1062858801516597, 40.86394065090267702, 12.00000000000001066 ) ) ;
#2340=AXIS2_PLACEMENT_3D ( 'NONE', #4332, #4572, #8066 ) ;
#2345=FACE_BOUND ( 'NONE', #12155, .T. ) ;
#2346=LINE ( 'NONE', #13458, #12195 ) ;
#2354=DIRECTION ( 'NONE',  ( -0.000000000000000000, 0.000000000000000000, 1.000000000000000000 ) ) ;
#2358=CARTESIAN_POINT ( 'NONE',  ( 114.0000000000000568, 59.53993994372674337, 15.00000000000035172 ) ) ;
#2359=CIRCLE ( 'NONE', #7167, 1.499999999999994449 ) ;
#2361=FILL_AREA_STYLE_COLOUR ( '', #312 ) ;
#2365=VECTOR ( 'NONE', #14176, 1000.000000000000000 ) ;
#2371=EDGE_CURVE ( 'NONE', #3949, #591, #8596, .T. ) ;
#2373=CARTESIAN_POINT ( 'NONE',  ( 224.0000000000000853, 56.53993994372675047, 13.00000000000000178 ) ) ;
#2382=ORIENTED_EDGE ( 'NONE', *, *, #8690, .F. ) ;
#2385=CARTESIAN_POINT ( 'NONE',  ( -76.50000000000001421, 17.53993994372674692, -17.50000000000002487 ) ) ;
#2389=ORIENTED_EDGE ( 'NONE', *, *, #13377, .F. ) ;
#2395=ORIENTED_EDGE ( 'NONE', *, *, #5493, .F. ) ;
#2401=FACE_OUTER_BOUND ( 'NONE', #10998, .T. ) ;
#2402=ADVANCED_FACE ( 'NONE', ( #9396, #5612 ), #4334, .F. ) ;
#2404=EDGE_LOOP ( 'NONE', ( #11306, #9340, #9210, #49 ) ) ;
#2411=DIRECTION ( 'NONE',  ( 0.000000000000000000, 1.156482317317871725E-16, -1.000000000000000000 ) ) ;
#2412=VERTEX_POINT ( 'NONE', #774 ) ;
#2414=DIRECTION ( 'NONE',  ( 0.000000000000000000, -1.000000000000000000, -1.486905836551548832E-16 ) ) ;
#2418=ORIENTED_EDGE ( 'NONE', *, *, #3717, .T. ) ;
#2427=DIRECTION ( 'NONE',  ( -0.000000000000000000, 1.000000000000000000, 0.000000000000000000 ) ) ;
#2435=ORIENTED_EDGE ( 'NONE', *, *, #7859, .F. ) ;
#2436=CARTESIAN_POINT ( 'NONE',  ( -85.99999999999994316, 64.53993994372673626, 11.50000000000174438 ) ) ;
#2442=DIRECTION ( 'NONE',  ( -0.000000000000000000, 1.000000000000000000, -0.000000000000000000 ) ) ;
#2450=ORIENTED_EDGE ( 'NONE', *, *, #10508, .F. ) ;
#2455=DIRECTION ( 'NONE',  ( -0.000000000000000000, -1.000000000000000000, -0.000000000000000000 ) ) ;
#2456=CARTESIAN_POINT ( 'NONE',  ( -35.99999999999995026, 59.53993994372674337, 15.00000000000139977 ) ) ;
#2460=CARTESIAN_POINT ( 'NONE',  ( 164.0000000000000568, 64.53993994372673626, 18.52500000000000213 ) ) ;
#2462=ORIENTED_EDGE ( 'NONE', *, *, #12399, .F. ) ;
#2468=ORIENTED_EDGE ( 'NONE', *, *, #6146, .F. ) ;
#2472=ORIENTED_EDGE ( 'NONE', *, *, #12766, .F. ) ;
#2476=ADVANCED_FACE ( 'NONE', ( #3546, #1093 ), #1246, .F. ) ;
#2477=ADVANCED_FACE ( 'NONE', ( #10974, #11918 ), #8528, .F. ) ;
#2481=VECTOR ( 'NONE', #2055, 1000.000000000000000 ) ;
#2482=AXIS2_PLACEMENT_3D ( 'NONE', #12280, #12364, #11576 ) ;
#2483=DIRECTION ( 'NONE',  ( 0.000000000000000000, 0.000000000000000000, 1.000000000000000000 ) ) ;
#2490=VERTEX_POINT ( 'NONE', #55 ) ;
#2492=CARTESIAN_POINT ( 'NONE',  ( 0.000000000000000000, 19.53993994372674337, 2.905405074819403421E-15 ) ) ;
#2500=CARTESIAN_POINT ( 'NONE',  ( -63.50000000000002842, 17.53993994372673271, 52.49999999999997868 ) ) ;
#2507=EDGE_CURVE ( 'NONE', #11511, #6265, #10735, .T. ) ;
#2508=DIRECTION ( 'NONE',  ( 0.000000000000000000, 0.000000000000000000, 1.000000000000000000 ) ) ;
#2517=VECTOR ( 'NONE', #6749, 1000.000000000000000 ) ;
#2522=CARTESIAN_POINT ( 'NONE',  ( -108.0000000000000568, 64.53993994372673626, 10.00000000000000178 ) ) ;
#2527=EDGE_LOOP ( 'NONE', ( #2811, #5685, #13665, #9298 ) ) ;
#2529=EDGE_CURVE ( 'NONE', #3509, #4053, #4812, .T. ) ;
#2541=AXIS2_PLACEMENT_3D ( 'NONE', #4583, #12869, #12947 ) ;
#2543=DIRECTION ( 'NONE',  ( 0.000000000000000000, 1.000000000000000000, 0.000000000000000000 ) ) ;
#2548=CIRCLE ( 'NONE', #11377, 1.700000000000007061 ) ;
#2550=ORIENTED_EDGE ( 'NONE', *, *, #4683, .T. ) ;
#2551=DIRECTION ( 'NONE',  ( 0.000000000000000000, -1.000000000000000000, 0.000000000000000000 ) ) ;
#2553=EDGE_CURVE ( 'NONE', #299, #9986, #9713, .T. ) ;
#2555=ORIENTED_EDGE ( 'NONE', *, *, #2553, .T. ) ;
#2574=ADVANCED_FACE ( 'NONE', ( #12221 ), #357, .F. ) ;
#2587=VECTOR ( 'NONE', #6441, 1000.000000000000000 ) ;
#2588=DIRECTION ( 'NONE',  ( -0.000000000000000000, 1.000000000000000000, -0.000000000000000000 ) ) ;
#2589=VECTOR ( 'NONE', #4836, 1000.000000000000000 ) ;
#2591=EDGE_CURVE ( 'NONE', #6470, #4243, #5199, .T. ) ;
#2592=DIRECTION ( 'NONE',  ( -0.000000000000000000, 1.000000000000000000, -0.000000000000000000 ) ) ;
#2601=CIRCLE ( 'NONE', #13674, 1.699999999999994849 ) ;
#2604=ORIENTED_EDGE ( 'NONE', *, *, #8057, .T. ) ;
#2605=VECTOR ( 'NONE', #3466, 1000.000000000000000 ) ;
#2607=DIRECTION ( 'NONE',  ( -0.000000000000000000, -0.000000000000000000, 1.000000000000000000 ) ) ;
#2610=EDGE_LOOP ( 'NONE', ( #6247, #8856 ) ) ;
#2611=AXIS2_PLACEMENT_3D ( 'NONE', #7905, #841, #9307 ) ;
#2613=EDGE_LOOP ( 'NONE', ( #2450, #9720, #11799, #2764 ) ) ;
#2614=DIRECTION ( 'NONE',  ( -0.000000000000000000, 1.000000000000000000, 1.156482317317871725E-16 ) ) ;
#2616=( GEOMETRIC_REPRESENTATION_CONTEXT ( 3 ) GLOBAL_UNCERTAINTY_ASSIGNED_CONTEXT ( ( #4060 ) ) GLOBAL_UNIT_ASSIGNED_CONTEXT ( ( #12452, #13713, #2835 ) ) REPRESENTATION_CONTEXT ( 'NONE', 'WORKASPACE' ) );
#2620=LINE ( 'NONE', #12470, #1574 ) ;
#2621=EDGE_LOOP ( 'NONE', ( #1993, #8913 ) ) ;
#2623=EDGE_CURVE ( 'NONE', #6805, #5504, #3445, .T. ) ;
#2627=LINE ( 'NONE', #7376, #597 ) ;
#2629=ORIENTED_EDGE ( 'NONE', *, *, #2176, .T. ) ;
#2636=ORIENTED_EDGE ( 'NONE', *, *, #10806, .F. ) ;
#2637=VECTOR ( 'NONE', #300, 1000.000000000000000 ) ;
#2638=CARTESIAN_POINT ( 'NONE',  ( -85.99999999999994316, 64.53993994372673626, 15.00000000000174794 ) ) ;
#2639=CARTESIAN_POINT ( 'NONE',  ( -108.0000000000000568, 59.53993994372674337, 10.00000000000000178 ) ) ;
#2642=EDGE_CURVE ( 'NONE', #2137, #5720, #8838, .T. ) ;
#2644=FACE_BOUND ( 'NONE', #4039, .T. ) ;
#2650=CARTESIAN_POINT ( 'NONE',  ( 177.5000000000000853, 17.53993994372673271, 52.49999999999997868 ) ) ;
#2661=EDGE_CURVE ( 'NONE', #10578, #8016, #14281, .T. ) ;
#2665=DIRECTION ( 'NONE',  ( 0.000000000000000000, 0.000000000000000000, 1.000000000000000000 ) ) ;
#2669=DIRECTION ( 'NONE',  ( -0.000000000000000000, 1.000000000000000000, -0.000000000000000000 ) ) ;
#2673=VERTEX_POINT ( 'NONE', #11277 ) ;
#2683=EDGE_CURVE ( 'NONE', #10665, #2814, #929, .T. ) ;
#2693=CARTESIAN_POINT ( 'NONE',  ( -110.0000000000000426, 22.53993994372673981, 13.00000000000000178 ) ) ;
#2695=AXIS2_PLACEMENT_3D ( 'NONE', #7638, #1622, #11110 ) ;
#2703=CARTESIAN_POINT ( 'NONE',  ( -110.0000000000000426, 19.53993994372674337, 9.999999999999998224 ) ) ;
#2714=DIRECTION ( 'NONE',  ( -0.000000000000000000, 1.000000000000000000, -0.000000000000000000 ) ) ;
#2716=LINE ( 'NONE', #5086, #1760 ) ;
#2718=LINE ( 'NONE', #4934, #2587 ) ;
#2719=EDGE_CURVE ( 'NONE', #591, #3949, #6727, .T. ) ;
#2727=ORIENTED_EDGE ( 'NONE', *, *, #9676, .F. ) ;
#2750=ORIENTED_EDGE ( 'NONE', *, *, #5008, .F. ) ;
#2751=EDGE_LOOP ( 'NONE', ( #250, #275, #8439, #15379 ) ) ;
#2755=DIRECTION ( 'NONE',  ( -0.000000000000000000, 1.000000000000000000, -0.000000000000000000 ) ) ;
#2764=ORIENTED_EDGE ( 'NONE', *, *, #13266, .T. ) ;
#2765=AXIS2_PLACEMENT_3D ( 'NONE', #2957, #7779, #12567 ) ;
#2771=EDGE_LOOP ( 'NONE', ( #6205, #9640, #7848, #6477 ) ) ;
#2781=VECTOR ( 'NONE', #11909, 1000.000000000000000 ) ;
#2782=CONICAL_SURFACE ( 'NONE', #10587, 3.524999999999998579, 0.7853981633974482790 ) ;
#2784=ORIENTED_EDGE ( 'NONE', *, *, #7217, .T. ) ;
#2803=CONICAL_SURFACE ( 'NONE', #2289, 3.525000000000000355, 0.7853981633974482790 ) ;
#2804=EDGE_CURVE ( 'NONE', #2947, #6121, #12506, .T. ) ;
#2805=PLANE ( 'NONE',  #14917 ) ;
#2806=VERTEX_POINT ( 'NONE', #4709 ) ;
#2811=ORIENTED_EDGE ( 'NONE', *, *, #1880, .F. ) ;
#2814=VERTEX_POINT ( 'NONE', #2264 ) ;
#2815=VECTOR ( 'NONE', #12122, 1000.000000000000000 ) ;
#2823=CIRCLE ( 'NONE', #1287, 1.699999999999996625 ) ;
#2824=DIRECTION ( 'NONE',  ( 0.000000000000000000, -1.000000000000000000, -1.156482317317871478E-16 ) ) ;
#2830=CARTESIAN_POINT ( 'NONE',  ( 64.00000000000005684, 59.53993994372674337, 15.00000000000070166 ) ) ;
#2833=PLANE ( 'NONE',  #5632 ) ;
#2834=CARTESIAN_POINT ( 'NONE',  ( 184.0000000000000568, 17.53993994372673271, 48.99999999999997158 ) ) ;
#2835=( NAMED_UNIT ( * ) SI_UNIT ( $, .STERADIAN. ) SOLID_ANGLE_UNIT ( ) );
#2840=AXIS2_PLACEMENT_3D ( 'NONE', #9711, #4723, #3545 ) ;
#2849=EDGE_LOOP ( 'NONE', ( #8044, #1302, #12370, #2119 ) ) ;
#2850=CARTESIAN_POINT ( 'NONE',  ( 184.0000000000000568, 17.53993994372673981, -12.49999999999999467 ) ) ;
#2856=ADVANCED_FACE ( 'NONE', ( #7256 ), #10005, .T. ) ;
#2867=CARTESIAN_POINT ( 'NONE',  ( 194.0000000000000568, 59.53993994372674337, 20.00000000000000355 ) ) ;
#2871=ORIENTED_EDGE ( 'NONE', *, *, #4683, .F. ) ;
#2875=DIRECTION ( 'NONE',  ( -0.000000000000000000, 1.000000000000000000, 0.000000000000000000 ) ) ;
#2877=CARTESIAN_POINT ( 'NONE',  ( -108.0000000000000568, 59.53993994372674337, 20.00000000000000355 ) ) ;
#2880=EDGE_CURVE ( 'NONE', #14289, #6589, #991, .T. ) ;
#2900=DIRECTION ( 'NONE',  ( 0.000000000000000000, 0.000000000000000000, 1.000000000000000000 ) ) ;
#2901=CARTESIAN_POINT ( 'NONE',  ( -35.99999999999995026, 64.53993994372673626, 15.00000000000139977 ) ) ;
#2902=EDGE_LOOP ( 'NONE', ( #10350, #2462 ) ) ;
#2903=DIRECTION ( 'NONE',  ( -0.000000000000000000, -0.000000000000000000, -1.000000000000000000 ) ) ;
#2907=EDGE_LOOP ( 'NONE', ( #5248, #13337, #5877, #13560 ) ) ;
#2908=DIRECTION ( 'NONE',  ( 0.000000000000000000, 0.000000000000000000, -1.000000000000000000 ) ) ;
#2911=EDGE_CURVE ( 'NONE', #5528, #12980, #7333, .T. ) ;
#2912=VERTEX_POINT ( 'NONE', #8215 ) ;
#2915=CARTESIAN_POINT ( 'NONE',  ( 224.0000000000000853, 59.53993994372674337, 25.00000000000000000 ) ) ;
#2916=CARTESIAN_POINT ( 'NONE',  ( 14.00000000000004086, 64.53993994372673626, 18.50000000000105160 ) ) ;
#2917=DIRECTION ( 'NONE',  ( 0.000000000000000000, 0.000000000000000000, 1.000000000000000000 ) ) ;
#2919=ORIENTED_EDGE ( 'NONE', *, *, #11934, .T. ) ;
#2947=VERTEX_POINT ( 'NONE', #13532 ) ;
#2949=DIRECTION ( 'NONE',  ( -1.000000000000000000, 0.000000000000000000, 0.000000000000000000 ) ) ;
#2951=ORIENTED_EDGE ( 'NONE', *, *, #5707, .T. ) ;
#2953=FACE_OUTER_BOUND ( 'NONE', #8679, .T. ) ;
#2955=CYLINDRICAL_SURFACE ( 'NONE', #8999, 1.700000000000001954 ) ;
#2957=CARTESIAN_POINT ( 'NONE',  ( 224.0000000000000853, 26.39124795404934076, 0.000000000000000000 ) ) ;
#2960=DIRECTION ( 'NONE',  ( 1.000000000000000000, 0.000000000000000000, 0.000000000000000000 ) ) ;
#2966=ORIENTED_EDGE ( 'NONE', *, *, #13201, .F. ) ;
#2977=DIRECTION ( 'NONE',  ( 0.000000000000000000, 0.000000000000000000, 1.000000000000000000 ) ) ;
#2978=DIRECTION ( 'NONE',  ( 0.000000000000000000, 0.000000000000000000, 1.000000000000000000 ) ) ;
#2985=DIRECTION ( 'NONE',  ( -1.000000000000000000, -0.000000000000000000, 0.000000000000000000 ) ) ;
#2986=CARTESIAN_POINT ( 'NONE',  ( 194.0000000000000568, 64.53993994372673626, 10.00000000000000178 ) ) ;
#2988=CIRCLE ( 'NONE', #2482, 6.999999999999992006 ) ;
#2994=CARTESIAN_POINT ( 'NONE',  ( 185.1062858801516882, 25.86394065090268057, 18.00000000000000355 ) ) ;
#3003=DIRECTION ( 'NONE',  ( -0.000000000000000000, 1.486905836551548832E-16, -1.000000000000000000 ) ) ;
#3004=ORIENTED_EDGE ( 'NONE', *, *, #7863, .F. ) ;
#3006=DIRECTION ( 'NONE',  ( 0.000000000000000000, 0.000000000000000000, 1.000000000000000000 ) ) ;
#3012=ORIENTED_EDGE ( 'NONE', *, *, #11091, .F. ) ;
#3030=STYLED_ITEM ( 'NONE', ( #5938 ), #11070 ) ;
#3032=FACE_OUTER_BOUND ( 'NONE', #1952, .T. ) ;
#3033=CARTESIAN_POINT ( 'NONE',  ( 200.1062858801516597, 40.86394065090267702, 18.00000000000000355 ) ) ;
#3036=DIRECTION ( 'NONE',  ( 0.000000000000000000, 0.000000000000000000, 1.000000000000000000 ) ) ;
#3042=FACE_OUTER_BOUND ( 'NONE', #467, .T. ) ;
#3050=EDGE_CURVE ( 'NONE', #11465, #4254, #14521, .T. ) ;
#3051=CARTESIAN_POINT ( 'NONE',  ( 185.1062858801516882, 25.86394065090268057, 13.00000000000000178 ) ) ;
#3055=EDGE_LOOP ( 'NONE', ( #12716, #12912, #8, #6125 ) ) ;
#3061=VERTEX_POINT ( 'NONE', #413 ) ;
#3067=DIRECTION ( 'NONE',  ( 0.000000000000000000, -1.000000000000000000, -1.156482317317871478E-16 ) ) ;
#3071=CARTESIAN_POINT ( 'NONE',  ( -110.0000000000000426, 59.53993994372674337, 10.00000000000000178 ) ) ;
#3080=ORIENTED_EDGE ( 'NONE', *, *, #15415, .T. ) ;
#3082=EDGE_LOOP ( 'NONE', ( #14976, #4117, #13374, #3753 ) ) ;
#3091=ORIENTED_EDGE ( 'NONE', *, *, #14050, .T. ) ;
#3100=ORIENTED_EDGE ( 'NONE', *, *, #9245, .F. ) ;
#3107=DIRECTION ( 'NONE',  ( 0.000000000000000000, 0.000000000000000000, 1.000000000000000000 ) ) ;
#3111=LINE ( 'NONE', #13838, #2517 ) ;
#3113=DIRECTION ( 'NONE',  ( 0.000000000000000000, 0.000000000000000000, -1.000000000000000000 ) ) ;
#3120=AXIS2_PLACEMENT_3D ( 'NONE', #12292, #1245, #6314 ) ;
#3124=AXIS2_PLACEMENT_3D ( 'NONE', #11439, #1646, #7665 ) ;
#3129=DIRECTION ( 'NONE',  ( 0.000000000000000000, 0.000000000000000000, 1.000000000000000000 ) ) ;
#3130=DIRECTION ( 'NONE',  ( -0.000000000000000000, 1.000000000000000000, -0.000000000000000000 ) ) ;
#3136=CARTESIAN_POINT ( 'NONE',  ( 177.5000000000000853, 19.53993994372674692, -17.50000000000002487 ) ) ;
#3137=LINE ( 'NONE', #7895, #5238 ) ;
#3139=EDGE_CURVE ( 'NONE', #9730, #5113, #11517, .T. ) ;
#3143=DIRECTION ( 'NONE',  ( -0.000000000000000000, 1.000000000000000000, -0.000000000000000000 ) ) ;
#3144=CARTESIAN_POINT ( 'NONE',  ( -110.0000000000000426, 22.53993994372673981, 13.00000000000000178 ) ) ;
#3147=AXIS2_PLACEMENT_3D ( 'NONE', #8822, #2824, #2665 ) ;
#3149=ORIENTED_EDGE ( 'NONE', *, *, #3532, .T. ) ;
#3170=DIRECTION ( 'NONE',  ( -0.000000000000000000, 1.000000000000000000, -0.000000000000000000 ) ) ;
#3171=ORIENTED_EDGE ( 'NONE', *, *, #1484, .T. ) ;
#3179=CYLINDRICAL_SURFACE ( 'NONE', #13769, 1.499999999999994449 ) ;
#3180=CYLINDRICAL_SURFACE ( 'NONE', #7074, 5.000000000000004441 ) ;
#3181=AXIS2_PLACEMENT_3D ( 'NONE', #8514, #6140, #4789 ) ;
#3182=CARTESIAN_POINT ( 'NONE',  ( 224.0000000000000853, 59.53993994372674337, 25.00000000000000000 ) ) ;
#3194=DIRECTION ( 'NONE',  ( -0.000000000000000000, 1.000000000000000000, 0.000000000000000000 ) ) ;
#3204=DIRECTION ( 'NONE',  ( -0.000000000000000000, 1.156482317317871478E-16, -1.000000000000000000 ) ) ;
#3205=ORIENTED_EDGE ( 'NONE', *, *, #2553, .F. ) ;
#3208=ORIENTED_EDGE ( 'NONE', *, *, #12766, .T. ) ;
#3215=EDGE_CURVE ( 'NONE', #10303, #5951, #13758, .T. ) ;
#3225=AXIS2_PLACEMENT_3D ( 'NONE', #13000, #14185, #5466 ) ;
#3232=PRODUCT_DEFINITION_SHAPE ( 'NONE', 'NONE',  #15380 ) ;
#3241=FACE_BOUND ( 'NONE', #13785, .T. ) ;
#3246=ADVANCED_FACE ( 'NONE', ( #15412, #14235, #3659, #4686, #9438, #10860, #12031 ), #4532, .T. ) ;
#3266=DIRECTION ( 'NONE',  ( 0.000000000000000000, -1.000000000000000000, 0.000000000000000000 ) ) ;
#3271=AXIS2_PLACEMENT_3D ( 'NONE', #4361, #1683, #12650 ) ;
#3272=EDGE_CURVE ( 'NONE', #2490, #1161, #9511, .T. ) ;
#3273=ORIENTED_EDGE ( 'NONE', *, *, #36, .F. ) ;
#3279=EDGE_CURVE ( 'NONE', #435, #9262, #14, .T. ) ;
#3287=FACE_OUTER_BOUND ( 'NONE', #14716, .T. ) ;
#3291=ORIENTED_EDGE ( 'NONE', *, *, #5066, .F. ) ;
#3294=ORIENTED_EDGE ( 'NONE', *, *, #2591, .F. ) ;
#3308=VECTOR ( 'NONE', #10953, 1000.000000000000114 ) ;
#3309=DIRECTION ( 'NONE',  ( -0.000000000000000000, 1.000000000000000000, -0.000000000000000000 ) ) ;
#3312=ORIENTED_EDGE ( 'NONE', *, *, #9621, .T. ) ;
#3334=ORIENTED_EDGE ( 'NONE', *, *, #1545, .T. ) ;
#3336=LINE ( 'NONE', #12718, #5801 ) ;
#3343=CARTESIAN_POINT ( 'NONE',  ( 177.5000000000000853, 17.53993994372674692, -17.50000000000002487 ) ) ;
#3346=LINE ( 'NONE', #8330, #13366 ) ;
#3347=CARTESIAN_POINT ( 'NONE',  ( 184.0000000000000568, 19.53993994372673626, 45.99999999999998579 ) ) ;
#3348=ORIENTED_EDGE ( 'NONE', *, *, #11478, .F. ) ;
#3355=CARTESIAN_POINT ( 'NONE',  ( 185.1062858801516597, 25.86394065090268057, 13.00000000000000178 ) ) ;
#3373=CARTESIAN_POINT ( 'NONE',  ( 114.0000000000000568, 62.13993994372673768, 15.00000000000035172 ) ) ;
#3375=DIRECTION ( 'NONE',  ( -0.000000000000000000, 1.000000000000000000, 8.673617379884035472E-17 ) ) ;
#3383=EDGE_CURVE ( 'NONE', #4243, #61, #11087, .T. ) ;
#3395=DIRECTION ( 'NONE',  ( 0.000000000000000000, 0.000000000000000000, 1.000000000000000000 ) ) ;
#3396=ORIENTED_EDGE ( 'NONE', *, *, #10958, .T. ) ;
#3397=VECTOR ( 'NONE', #12363, 1000.000000000000000 ) ;
#3398=EDGE_CURVE ( 'NONE', #3061, #15478, #3899, .T. ) ;
#3399=ORIENTED_EDGE ( 'NONE', *, *, #10257, .T. ) ;
#3403=CYLINDRICAL_SURFACE ( 'NONE', #3429, 1.699999999999991518 ) ;
#3406=ORIENTED_EDGE ( 'NONE', *, *, #6142, .F. ) ;
#3407=ORIENTED_EDGE ( 'NONE', *, *, #15254, .T. ) ;
#3414=DIRECTION ( 'NONE',  ( -0.000000000000000000, 1.000000000000000000, -0.000000000000000000 ) ) ;
#3429=AXIS2_PLACEMENT_3D ( 'NONE', #4736, #1024, #9560 ) ;
#3430=DIRECTION ( 'NONE',  ( 1.000000000000000000, 0.000000000000000000, 0.000000000000000000 ) ) ;
#3434=ORIENTED_EDGE ( 'NONE', *, *, #4211, .F. ) ;
#3437=EDGE_LOOP ( 'NONE', ( #3714, #6625 ) ) ;
#3439=ADVANCED_FACE ( 'NONE', ( #14540 ), #5236, .F. ) ;
#3441=DIRECTION ( 'NONE',  ( -0.000000000000000000, 1.000000000000000000, 1.486905836551548832E-16 ) ) ;
#3445=CIRCLE ( 'NONE', #5468, 3.525000000000002132 ) ;
#3458=CARTESIAN_POINT ( 'NONE',  ( -35.99999999999995026, 64.53993994372673626, 15.00000000000139977 ) ) ;
#3466=DIRECTION ( 'NONE',  ( -1.000000000000000000, -0.000000000000000000, -0.000000000000000000 ) ) ;
#3472=ORIENTED_EDGE ( 'NONE', *, *, #3139, .T. ) ;
#3475=CARTESIAN_POINT ( 'NONE',  ( 14.00000000000004086, 64.53993994372673626, 18.52500000000105018 ) ) ;
#3489=VECTOR ( 'NONE', #5079, 1000.000000000000000 ) ;
#3492=ORIENTED_EDGE ( 'NONE', *, *, #2047, .F. ) ;
#3498=ORIENTED_EDGE ( 'NONE', *, *, #9348, .T. ) ;
#3502=ORIENTED_EDGE ( 'NONE', *, *, #2661, .T. ) ;
#3509=VERTEX_POINT ( 'NONE', #13592 ) ;
#3522=EDGE_LOOP ( 'NONE', ( #15265, #15251 ) ) ;
#3524=FACE_BOUND ( 'NONE', #2902, .T. ) ;
#3532=EDGE_CURVE ( 'NONE', #6607, #8299, #1601, .T. ) ;
#3536=DIRECTION ( 'NONE',  ( 1.000000000000000000, 0.000000000000000000, 0.000000000000000000 ) ) ;
#3540=PLANE ( 'NONE',  #13909 ) ;
#3542=ORIENTED_EDGE ( 'NONE', *, *, #5274, .T. ) ;
#3545=DIRECTION ( 'NONE',  ( 0.000000000000000000, 0.000000000000000000, 1.000000000000000000 ) ) ;
#3546=FACE_BOUND ( 'NONE', #4034, .T. ) ;
#3549=ADVANCED_FACE ( 'NONE', ( #14931 ), #2955, .F. ) ;
#3552=VERTEX_POINT ( 'NONE', #6515 ) ;
#3558=DIRECTION ( 'NONE',  ( 0.000000000000000000, 0.000000000000000000, 1.000000000000000000 ) ) ;
#3565=ADVANCED_FACE ( 'NONE', ( #7774 ), #3179, .F. ) ;
#3570=DIRECTION ( 'NONE',  ( 0.000000000000000000, 0.000000000000000000, 1.000000000000000000 ) ) ;
#3580=ORIENTED_EDGE ( 'NONE', *, *, #13086, .F. ) ;
#3585=ORIENTED_EDGE ( 'NONE', *, *, #2661, .F. ) ;
#3612=CYLINDRICAL_SURFACE ( 'NONE', #1091, 5.000000000000004441 ) ;
#3614=CIRCLE ( 'NONE', #7185, 1.700000000000001954 ) ;
#3615=FACE_OUTER_BOUND ( 'NONE', #10833, .T. ) ;
#3626=CARTESIAN_POINT ( 'NONE',  ( -35.99999999999995026, 64.53993994372673626, 18.52500000000140190 ) ) ;
#3630=CIRCLE ( 'NONE', #14201, 1.700000000000007061 ) ;
#3633=ADVANCED_FACE ( 'NONE', ( #3032 ), #7937, .T. ) ;
#3638=EDGE_LOOP ( 'NONE', ( #11666, #12162, #10756, #4770 ) ) ;
#3644=LINE ( 'NONE', #10843, #2589 ) ;
#3649=LINE ( 'NONE', #959, #1133 ) ;
#3654=EDGE_LOOP ( 'NONE', ( #4120, #5910, #4456, #3080 ) ) ;
#3659=FACE_BOUND ( 'NONE', #368, .T. ) ;
#3660=CARTESIAN_POINT ( 'NONE',  ( 64.00000000000005684, 64.53993994372673626, 11.47500000000070131 ) ) ;
#3662=EDGE_CURVE ( 'NONE', #435, #13457, #8012, .T. ) ;
#3672=EDGE_LOOP ( 'NONE', ( #6926, #303, #10523, #3929 ) ) ;
#3674=FACE_OUTER_BOUND ( 'NONE', #2771, .T. ) ;
#3680=CARTESIAN_POINT ( 'NONE',  ( 200.1062858801516597, 47.86394065090266992, 10.00000000000000533 ) ) ;
#3684=CARTESIAN_POINT ( 'NONE',  ( -110.0000000000000426, 19.53993994372674337, 24.99999999999999645 ) ) ;
#3688=CARTESIAN_POINT ( 'NONE',  ( 14.00000000000004086, 62.13993994372673768, 11.50000000000105160 ) ) ;
#3692=DIRECTION ( 'NONE',  ( 0.000000000000000000, 0.000000000000000000, 1.000000000000000000 ) ) ;
#3700=EDGE_CURVE ( 'NONE', #319, #6121, #5316, .T. ) ;
#3702=DIRECTION ( 'NONE',  ( -0.000000000000000000, 1.000000000000000000, -0.000000000000000000 ) ) ;
#3711=ORIENTED_EDGE ( 'NONE', *, *, #14847, .F. ) ;
#3714=ORIENTED_EDGE ( 'NONE', *, *, #8427, .F. ) ;
#3717=EDGE_CURVE ( 'NONE', #15409, #14286, #7742, .T. ) ;
#3722=EDGE_CURVE ( 'NONE', #14758, #8929, #4955, .T. ) ;
#3727=EDGE_LOOP ( 'NONE', ( #15081, #12045 ) ) ;
#3736=EDGE_LOOP ( 'NONE', ( #11688, #13847, #11326, #13585 ) ) ;
#3743=DIRECTION ( 'NONE',  ( 1.000000000000000000, 0.000000000000000000, 0.000000000000000000 ) ) ;
#3745=DIRECTION ( 'NONE',  ( -0.000000000000000000, 1.000000000000000000, -0.000000000000000000 ) ) ;
#3753=ORIENTED_EDGE ( 'NONE', *, *, #4567, .F. ) ;
#3766=VECTOR ( 'NONE', #7075, 1000.000000000000000 ) ;
#3770=DIRECTION ( 'NONE',  ( 0.000000000000000000, 0.000000000000000000, 1.000000000000000000 ) ) ;
#3773=ORIENTED_EDGE ( 'NONE', *, *, #6054, .T. ) ;
#3775=DIRECTION ( 'NONE',  ( 0.000000000000000000, 0.7071067811865474617, 0.7071067811865474617 ) ) ;
#3779=CIRCLE ( 'NONE', #6051, 2.000000000000001776 ) ;
#3786=ORIENTED_EDGE ( 'NONE', *, *, #2262, .T. ) ;
#3789=ORIENTED_EDGE ( 'NONE', *, *, #13568, .T. ) ;
#3799=EDGE_LOOP ( 'NONE', ( #7251, #8804, #7770, #8689 ) ) ;
#3806=SHAPE_REPRESENTATION ( 'Lower Fixed Bed Shear Blade', ( #12337 ), #4262 ) ;
#3808=ORIENTED_EDGE ( 'NONE', *, *, #5051, .T. ) ;
#3811=ORIENTED_EDGE ( 'NONE', *, *, #1313, .T. ) ;
#3816=EDGE_LOOP ( 'NONE', ( #4703, #15598 ) ) ;
#3817=VERTEX_POINT ( 'NONE', #391 ) ;
#3820=EDGE_CURVE ( 'NONE', #1161, #3061, #1516, .T. ) ;
#3834=CARTESIAN_POINT ( 'NONE',  ( -35.99999999999995026, 62.13993994372673768, 13.30000000000139870 ) ) ;
#3844=ORIENTED_EDGE ( 'NONE', *, *, #9771, .F. ) ;
#3852=EDGE_CURVE ( 'NONE', #10197, #13912, #236, .T. ) ;
#3861=CARTESIAN_POINT ( 'NONE',  ( 164.0000000000000568, 64.53993994372673626, 15.00000000000000355 ) ) ;
#3871=AXIS2_PLACEMENT_3D ( 'NONE', #8447, #15514, #3536 ) ;
#3876=VECTOR ( 'NONE', #9303, 1000.000000000000000 ) ;
#3883=AXIS2_PLACEMENT_3D ( 'NONE', #5256, #13696, #2900 ) ;
#3888=ORIENTED_EDGE ( 'NONE', *, *, #3383, .F. ) ;
#3896=AXIS2_PLACEMENT_3D ( 'NONE', #4839, #6186, #9813 ) ;
#3899=LINE ( 'NONE', #9828, #3926 ) ;
#3903=ORIENTED_EDGE ( 'NONE', *, *, #14111, .T. ) ;
#3904=CARTESIAN_POINT ( 'NONE',  ( 114.0000000000000568, 64.51493994372674479, 18.50000000000035527 ) ) ;
#3907=DIRECTION ( 'NONE',  ( 0.000000000000000000, 0.7071067811865474617, 0.7071067811865474617 ) ) ;
#3908=ORIENTED_EDGE ( 'NONE', *, *, #17, .T. ) ;
#3918=CARTESIAN_POINT ( 'NONE',  ( -63.50000000000002842, 17.53993994372674692, -17.50000000000002487 ) ) ;
#3923=LINE ( 'NONE', #116, #13312 ) ;
#3924=LINE ( 'NONE', #9863, #9146 ) ;
#3926=VECTOR ( 'NONE', #12256, 1000.000000000000000 ) ;
#3929=ORIENTED_EDGE ( 'NONE', *, *, #5008, .T. ) ;
#3944=ORIENTED_EDGE ( 'NONE', *, *, #5654, .F. ) ;
#3946=VERTEX_POINT ( 'NONE', #5702 ) ;
#3947=CARTESIAN_POINT ( 'NONE',  ( -35.99999999999995026, 62.13993994372673768, 11.50000000000139622 ) ) ;
#3949=VERTEX_POINT ( 'NONE', #5474 ) ;
#3955=VERTEX_POINT ( 'NONE', #8089 ) ;
#3986=DIRECTION ( 'NONE',  ( -0.000000000000000000, -0.000000000000000000, -1.000000000000000000 ) ) ;
#3990=CIRCLE ( 'NONE', #12816, 1.699999999999991518 ) ;
#3991=PLANE ( 'NONE',  #11807 ) ;
#3993=ORIENTED_EDGE ( 'NONE', *, *, #13266, .F. ) ;
#3998=ORIENTED_EDGE ( 'NONE', *, *, #625, .F. ) ;
#3999=CARTESIAN_POINT ( 'NONE',  ( 190.5000000000000568, 17.53993994372674692, -17.50000000000002487 ) ) ;
#4002=LINE ( 'NONE', #7579, #10686 ) ;
#4003=CARTESIAN_POINT ( 'NONE',  ( -108.0000000000000568, 59.53993994372674337, 10.00000000000000178 ) ) ;
#4015=AXIS2_PLACEMENT_3D ( 'NONE', #957, #4751, #8252 ) ;
#4024=EDGE_CURVE ( 'NONE', #5590, #10586, #7289, .T. ) ;
#4027=CARTESIAN_POINT ( 'NONE',  ( 177.5000000000000853, 19.53993994372674692, -17.50000000000002487 ) ) ;
#4034=EDGE_LOOP ( 'NONE', ( #10441, #8376 ) ) ;
#4039=EDGE_LOOP ( 'NONE', ( #10951, #8463 ) ) ;
#4047=CARTESIAN_POINT ( 'NONE',  ( -110.0000000000000426, 19.53993994372674337, 24.99999999999999645 ) ) ;
#4053=VERTEX_POINT ( 'NONE', #13910 ) ;
#4060=UNCERTAINTY_MEASURE_WITH_UNIT (LENGTH_MEASURE( 1.000000000000000082E-05 ), #12452, 'distance_accuracy_value', 'NONE');
#4067=DIRECTION ( 'NONE',  ( 0.000000000000000000, 0.000000000000000000, 1.000000000000000000 ) ) ;
#4080=ORIENTED_EDGE ( 'NONE', *, *, #8736, .T. ) ;
#4082=CARTESIAN_POINT ( 'NONE',  ( -85.99999999999994316, 64.53993994372673626, 15.00000000000174794 ) ) ;
#4083=DIRECTION ( 'NONE',  ( 1.000000000000000000, 0.000000000000000000, 0.000000000000000000 ) ) ;
#4085=DIRECTION ( 'NONE',  ( 0.000000000000000000, 0.000000000000000000, -1.000000000000000000 ) ) ;
#4087=CARTESIAN_POINT ( 'NONE',  ( 193.1062858801516882, 40.86394065090267702, 16.00000000000001421 ) ) ;
#4100=DIRECTION ( 'NONE',  ( 0.000000000000000000, 0.000000000000000000, 1.000000000000000000 ) ) ;
#4102=CARTESIAN_POINT ( 'NONE',  ( 205.1062858801516597, 40.86394065090267702, -219.0000000000000853 ) ) ;
#4108=EDGE_LOOP ( 'NONE', ( #9068, #2784, #315, #15001 ) ) ;
#4117=ORIENTED_EDGE ( 'NONE', *, *, #10392, .F. ) ;
#4119=DIRECTION ( 'NONE',  ( -0.000000000000000000, 1.000000000000000000, -0.000000000000000000 ) ) ;
#4120=ORIENTED_EDGE ( 'NONE', *, *, #9571, .F. ) ;
#4128=CARTESIAN_POINT ( 'NONE',  ( -35.99999999999995026, 59.53993994372674337, 15.00000000000139977 ) ) ;
#4136=VECTOR ( 'NONE', #2455, 1000.000000000000000 ) ;
#4138=CARTESIAN_POINT ( 'NONE',  ( -110.0000000000000426, 59.53993994372674337, 25.00000000000000000 ) ) ;
#4140=EDGE_CURVE ( 'NONE', #4254, #4264, #1108, .T. ) ;
#4143=DIRECTION ( 'NONE',  ( 0.000000000000000000, -1.486905836551548832E-16, 1.000000000000000000 ) ) ;
#4150=DIRECTION ( 'NONE',  ( 0.000000000000000000, 0.000000000000000000, -1.000000000000000000 ) ) ;
#4159=CARTESIAN_POINT ( 'NONE',  ( 200.1062858801516597, 40.86394065090267702, 12.00000000000001066 ) ) ;
#4162=CYLINDRICAL_SURFACE ( 'NONE', #7935, 1.700000000000007061 ) ;
#4164=EDGE_CURVE ( 'NONE', #10243, #5947, #10062, .T. ) ;
#4171=DIRECTION ( 'NONE',  ( 0.000000000000000000, -1.000000000000000000, 0.000000000000000000 ) ) ;
#4180=ORIENTED_EDGE ( 'NONE', *, *, #422, .F. ) ;
#4186=ORIENTED_EDGE ( 'NONE', *, *, #2371, .F. ) ;
#4188=DIRECTION ( 'NONE',  ( 0.000000000000000000, -1.486905836551548832E-16, 1.000000000000000000 ) ) ;
#4191=ORIENTED_EDGE ( 'NONE', *, *, #11111, .F. ) ;
#4199=VECTOR ( 'NONE', #7498, 1000.000000000000000 ) ;
#4211=EDGE_CURVE ( 'NONE', #9404, #6055, #6176, .T. ) ;
#4217=ADVANCED_FACE ( 'NONE', ( #4662 ), #8318, .F. ) ;
#4218=FACE_OUTER_BOUND ( 'NONE', #10868, .T. ) ;
#4223=CARTESIAN_POINT ( 'NONE',  ( 184.0000000000000568, 17.53993994372673981, -12.49999999999999467 ) ) ;
#4224=EDGE_LOOP ( 'NONE', ( #5100, #4732, #4988, #5158, #14208 ) ) ;
#4231=DIRECTION ( 'NONE',  ( 0.000000000000000000, 0.000000000000000000, 1.000000000000000000 ) ) ;
#4243=VERTEX_POINT ( 'NONE', #1573 ) ;
#4253=FACE_OUTER_BOUND ( 'NONE', #1938, .T. ) ;
#4254=VERTEX_POINT ( 'NONE', #3947 ) ;
#4262=( GEOMETRIC_REPRESENTATION_CONTEXT ( 3 ) GLOBAL_UNCERTAINTY_ASSIGNED_CONTEXT ( ( #5792 ) ) GLOBAL_UNIT_ASSIGNED_CONTEXT ( ( #5834, #14035, #2198 ) ) REPRESENTATION_CONTEXT ( 'NONE', 'WORKASPACE' ) );
#4264=VERTEX_POINT ( 'NONE', #13563 ) ;
#4268=DIRECTION ( 'NONE',  ( 0.000000000000000000, -1.000000000000000000, 0.000000000000000000 ) ) ;
#4271=DIRECTION ( 'NONE',  ( -0.000000000000000000, 1.000000000000000000, -0.000000000000000000 ) ) ;
#4278=FACE_BOUND ( 'NONE', #11004, .T. ) ;
#4286=CARTESIAN_POINT ( 'NONE',  ( 114.0000000000000568, 64.53993994372673626, 18.50000000000035527 ) ) ;
#4293=CARTESIAN_POINT ( 'NONE',  ( 64.00000000000005684, 62.13993994372673768, 15.00000000000070166 ) ) ;
#4294=CIRCLE ( 'NONE', #12107, 1.699999999999993072 ) ;
#4295=CARTESIAN_POINT ( 'NONE',  ( -85.99999999999994316, 64.53993994372673626, 15.00000000000174794 ) ) ;
#4297=CARTESIAN_POINT ( 'NONE',  ( 114.0000000000000568, 56.53993994372675047, 13.30000000000035776 ) ) ;
#4299=DIRECTION ( 'NONE',  ( 0.000000000000000000, 0.000000000000000000, 1.000000000000000000 ) ) ;
#4302=EDGE_CURVE ( 'NONE', #8562, #2806, #7556, .T. ) ;
#4311=VECTOR ( 'NONE', #7207, 1000.000000000000000 ) ;
#4312=CARTESIAN_POINT ( 'NONE',  ( -108.0000000000000568, 59.53993994372674337, 10.00000000000000178 ) ) ;
#4314=DIRECTION ( 'NONE',  ( -0.000000000000000000, 1.000000000000000000, -0.000000000000000000 ) ) ;
#4321=VECTOR ( 'NONE', #925, 1000.000000000000000 ) ;
#4328=ORIENTED_EDGE ( 'NONE', *, *, #5066, .T. ) ;
#4330=FACE_OUTER_BOUND ( 'NONE', #9823, .T. ) ;
#4332=CARTESIAN_POINT ( 'NONE',  ( 184.0000000000000568, 19.53993994372673626, 47.49999999999997868 ) ) ;
#4334=PLANE ( 'NONE',  #12762 ) ;
#4355=CARTESIAN_POINT ( 'NONE',  ( -35.99999999999995026, 64.53993994372673626, 13.30000000000139870 ) ) ;
#4361=CARTESIAN_POINT ( 'NONE',  ( 14.00000000000004086, 64.53993994372673626, 15.00000000000104983 ) ) ;
#4367=ORIENTED_EDGE ( 'NONE', *, *, #11357, .F. ) ;
#4370=CIRCLE ( 'NONE', #821, 1.699999999999993072 ) ;
#4371=ORIENTED_EDGE ( 'NONE', *, *, #13568, .F. ) ;
#4385=FACE_OUTER_BOUND ( 'NONE', #10020, .T. ) ;
#4390=ORIENTED_EDGE ( 'NONE', *, *, #4702, .F. ) ;
#4393=VECTOR ( 'NONE', #13658, 1000.000000000000000 ) ;
#4395=DIRECTION ( 'NONE',  ( 0.000000000000000000, 0.000000000000000000, 1.000000000000000000 ) ) ;
#4403=CYLINDRICAL_SURFACE ( 'NONE', #6157, 1.699999999999993072 ) ;
#4404=FACE_OUTER_BOUND ( 'NONE', #4224, .T. ) ;
#4422=CIRCLE ( 'NONE', #15504, 1.700000000000000178 ) ;
#4424=ORIENTED_EDGE ( 'NONE', *, *, #13659, .F. ) ;
#4428=CARTESIAN_POINT ( 'NONE',  ( 64.00000000000005684, 62.13993994372673768, 11.50000000000069811 ) ) ;
#4434=CARTESIAN_POINT ( 'NONE',  ( 185.1062858801516882, 55.86394065090267702, 18.00000000000000355 ) ) ;
#4438=FACE_OUTER_BOUND ( 'NONE', #1319, .T. ) ;
#4454=CARTESIAN_POINT ( 'NONE',  ( -85.99999999999994316, 62.13993994372673768, 16.70000000000174012 ) ) ;
#4456=ORIENTED_EDGE ( 'NONE', *, *, #14312, .T. ) ;
#4463=EDGE_CURVE ( 'NONE', #5113, #6601, #12142, .T. ) ;
#4466=CARTESIAN_POINT ( 'NONE',  ( -70.00000000000000000, 17.53993994372673981, -12.49999999999999467 ) ) ;
#4467=LINE ( 'NONE', #1940, #14058 ) ;
#4468=FACE_OUTER_BOUND ( 'NONE', #7347, .T. ) ;
#4478=DIRECTION ( 'NONE',  ( 1.000000000000000000, 0.000000000000000000, 0.000000000000000000 ) ) ;
#4480=CIRCLE ( 'NONE', #14302, 1.499999999999994449 ) ;
#4487=DIRECTION ( 'NONE',  ( -0.000000000000000000, 1.000000000000000000, -0.000000000000000000 ) ) ;
#4494=AXIS2_PLACEMENT_3D ( 'NONE', #11421, #12440, #13780 ) ;
#4511=ORIENTED_EDGE ( 'NONE', *, *, #10076, .T. ) ;
#4517=EDGE_CURVE ( 'NONE', #14978, #10303, #4888, .T. ) ;
#4518=DIRECTION ( 'NONE',  ( 0.000000000000000000, 0.000000000000000000, 1.000000000000000000 ) ) ;
#4527=CIRCLE ( 'NONE', #728, 1.700000000000001954 ) ;
#4532=PLANE ( 'NONE',  #12003 ) ;
#4537=ORIENTED_EDGE ( 'NONE', *, *, #5493, .T. ) ;
#4538=VECTOR ( 'NONE', #12198, 1000.000000000000000 ) ;
#4548=EDGE_LOOP ( 'NONE', ( #5605, #12232 ) ) ;
#4555=CARTESIAN_POINT ( 'NONE',  ( 114.0000000000000568, 64.51493994372674479, 15.00000000000035172 ) ) ;
#4559=DIRECTION ( 'NONE',  ( 0.000000000000000000, 0.000000000000000000, 1.000000000000000000 ) ) ;
#4562=CARTESIAN_POINT ( 'NONE',  ( -85.99999999999994316, 64.53993994372673626, 18.52500000000175007 ) ) ;
#4567=EDGE_CURVE ( 'NONE', #15158, #2814, #1734, .T. ) ;
#4568=CARTESIAN_POINT ( 'NONE',  ( 0.000000000000000000, 0.000000000000000000, 0.000000000000000000 ) ) ;
#4572=DIRECTION ( 'NONE',  ( 0.000000000000000000, -1.000000000000000000, -1.156482317317871478E-16 ) ) ;
#4582=CARTESIAN_POINT ( 'NONE',  ( 114.0000000000000568, 64.53993994372673626, 15.00000000000035172 ) ) ;
#4583=CARTESIAN_POINT ( 'NONE',  ( -70.00000000000000000, 17.53993994372673981, -12.49999999999999467 ) ) ;
#4584=CYLINDRICAL_SURFACE ( 'NONE', #7822, 3.500000000000004885 ) ;
#4594=CIRCLE ( 'NONE', #6116, 1.699999999999993072 ) ;
#4601=ORIENTED_EDGE ( 'NONE', *, *, #4674, .F. ) ;
#4609=AXIS2_PLACEMENT_3D ( 'NONE', #1470, #13709, #5267 ) ;
#4612=AXIS2_PLACEMENT_3D ( 'NONE', #3861, #13162, #11129 ) ;
#4614=VERTEX_POINT ( 'NONE', #7737 ) ;
#4619=CARTESIAN_POINT ( 'NONE',  ( -110.0000000000000426, 56.53993994372675047, 13.00000000000000178 ) ) ;
#4628=DIRECTION ( 'NONE',  ( 0.000000000000000000, 0.000000000000000000, 1.000000000000000000 ) ) ;
#4635=CIRCLE ( 'NONE', #14715, 1.499999999999997780 ) ;
#4638=DIRECTION ( 'NONE',  ( -0.000000000000000000, 1.000000000000000000, -0.000000000000000000 ) ) ;
#4639=DIRECTION ( 'NONE',  ( -0.000000000000000000, 1.000000000000000000, -0.000000000000000000 ) ) ;
#4657=DIRECTION ( 'NONE',  ( 0.000000000000000000, 0.000000000000000000, -1.000000000000000000 ) ) ;
#4658=FACE_OUTER_BOUND ( 'NONE', #8898, .T. ) ;
#4660=VERTEX_POINT ( 'NONE', #13474 ) ;
#4662=FACE_OUTER_BOUND ( 'NONE', #10271, .T. ) ;
#4674=EDGE_CURVE ( 'NONE', #8395, #6805, #6393, .T. ) ;
#4678=EDGE_LOOP ( 'NONE', ( #11411, #1684 ) ) ;
#4681=EDGE_LOOP ( 'NONE', ( #8358, #12568, #1905, #3903 ) ) ;
#4683=EDGE_CURVE ( 'NONE', #6607, #9401, #11041, .T. ) ;
#4686=FACE_BOUND ( 'NONE', #9424, .T. ) ;
#4694=VERTEX_POINT ( 'NONE', #6230 ) ;
#4695=CARTESIAN_POINT ( 'NONE',  ( 205.1062858801516597, 40.86394065090267702, 16.00000000000001421 ) ) ;
#4700=PLANE ( 'NONE',  #11134 ) ;
#4702=EDGE_CURVE ( 'NONE', #10245, #3061, #8833, .T. ) ;
#4703=ORIENTED_EDGE ( 'NONE', *, *, #14334, .T. ) ;
#4709=CARTESIAN_POINT ( 'NONE',  ( 114.0000000000000568, 59.53993994372674337, 16.70000000000034746 ) ) ;
#4713=CARTESIAN_POINT ( 'NONE',  ( -35.99999999999995026, 59.53993994372674337, 16.70000000000140261 ) ) ;
#4718=DIRECTION ( 'NONE',  ( 0.000000000000000000, 0.000000000000000000, 1.000000000000000000 ) ) ;
#4720=ORIENTED_EDGE ( 'NONE', *, *, #3717, .F. ) ;
#4723=DIRECTION ( 'NONE',  ( -0.000000000000000000, 1.000000000000000000, -0.000000000000000000 ) ) ;
#4729=VECTOR ( 'NONE', #7516, 1000.000000000000114 ) ;
#4731=VECTOR ( 'NONE', #8451, 1000.000000000000000 ) ;
#4732=ORIENTED_EDGE ( 'NONE', *, *, #5370, .T. ) ;
#4735=EDGE_LOOP ( 'NONE', ( #12519, #5855, #3773, #13655 ) ) ;
#4736=CARTESIAN_POINT ( 'NONE',  ( 64.00000000000005684, 64.53993994372673626, 15.00000000000070166 ) ) ;
#4741=PLANE ( 'NONE',  #14650 ) ;
#4746=CIRCLE ( 'NONE', #15313, 3.499999999999999556 ) ;
#4751=DIRECTION ( 'NONE',  ( -0.000000000000000000, 1.000000000000000000, 1.486905836551548832E-16 ) ) ;
#4756=AXIS2_PLACEMENT_3D ( 'NONE', #15342, #9450, #11664 ) ;
#4770=ORIENTED_EDGE ( 'NONE', *, *, #10039, .F. ) ;
#4775=VERTEX_POINT ( 'NONE', #2834 ) ;
#4780=FACE_OUTER_BOUND ( 'NONE', #8261, .T. ) ;
#4787=CARTESIAN_POINT ( 'NONE',  ( -108.0000000000000568, 59.53993994372674337, 10.00000000000000178 ) ) ;
#4789=DIRECTION ( 'NONE',  ( 0.000000000000000000, 0.000000000000000000, 1.000000000000000000 ) ) ;
#4797=EDGE_CURVE ( 'NONE', #14289, #11744, #8680, .T. ) ;
#4806=AXIS2_PLACEMENT_3D ( 'NONE', #10313, #15105, #13693 ) ;
#4812=LINE ( 'NONE', #1014, #10013 ) ;
#4815=EDGE_CURVE ( 'NONE', #259, #4660, #5667, .T. ) ;
#4818=CIRCLE ( 'NONE', #13384, 1.699999999999993072 ) ;
#4819=ORIENTED_EDGE ( 'NONE', *, *, #5843, .T. ) ;
#4821=LINE ( 'NONE', #2373, #4311 ) ;
#4822=ORIENTED_EDGE ( 'NONE', *, *, #10307, .F. ) ;
#4828=AXIS2_PLACEMENT_3D ( 'NONE', #1750, #14137, #9413 ) ;
#4835=EDGE_CURVE ( 'NONE', #4053, #1467, #10404, .T. ) ;
#4836=DIRECTION ( 'NONE',  ( 1.000000000000000000, 0.000000000000000000, 0.000000000000000000 ) ) ;
#4839=CARTESIAN_POINT ( 'NONE',  ( -35.99999999999995026, 64.53993994372673626, 15.00000000000139977 ) ) ;
#4856=CYLINDRICAL_SURFACE ( 'NONE', #2255, 1.699999999999996625 ) ;
#4857=EDGE_LOOP ( 'NONE', ( #2306, #11685, #11180, #10422 ) ) ;
#4871=ORIENTED_EDGE ( 'NONE', *, *, #5707, .F. ) ;
#4874=EDGE_CURVE ( 'NONE', #14286, #5616, #4467, .T. ) ;
#4880=CARTESIAN_POINT ( 'NONE',  ( 14.00000000000004086, 64.53993994372673626, 15.00000000000104983 ) ) ;
#4888=LINE ( 'NONE', #2436, #6542 ) ;
#4891=EDGE_CURVE ( 'NONE', #411, #868, #3137, .T. ) ;
#4899=EDGE_CURVE ( 'NONE', #5616, #5655, #13951, .T. ) ;
#4901=AXIS2_PLACEMENT_3D ( 'NONE', #11746, #6777, #10403 ) ;
#4903=AXIS2_PLACEMENT_3D ( 'NONE', #7979, #843, #9310 ) ;
#4904=CARTESIAN_POINT ( 'NONE',  ( -70.00000000000000000, 19.53993994372674337, -12.49999999999999467 ) ) ;
#4912=VERTEX_POINT ( 'NONE', #14097 ) ;
#4913=CARTESIAN_POINT ( 'NONE',  ( 177.5000000000000568, 19.53993994372674337, 24.99999999999999645 ) ) ;
#4914=LINE ( 'NONE', #7369, #14121 ) ;
#4915=TOROIDAL_SURFACE ( 'NONE', #9968, 6.999999999999991118, 2.000000000000000000 ) ;
#4922=EDGE_CURVE ( 'NONE', #2806, #8562, #11803, .T. ) ;
#4934=CARTESIAN_POINT ( 'NONE',  ( 114.0000000000000568, 64.53993994372673626, 16.70000000000034746 ) ) ;
#4942=EDGE_LOOP ( 'NONE', ( #546, #6060, #12457, #7673, #5946, #4390, #1148, #8475 ) ) ;
#4945=AXIS2_PLACEMENT_3D ( 'NONE', #2294, #12945, #4657 ) ;
#4946=ORIENTED_EDGE ( 'NONE', *, *, #10976, .F. ) ;
#4953=DIRECTION ( 'NONE',  ( 0.000000000000000000, 8.673617379884035472E-17, -1.000000000000000000 ) ) ;
#4955=CIRCLE ( 'NONE', #11011, 1.699999999999993072 ) ;
#4957=VECTOR ( 'NONE', #3375, 1000.000000000000000 ) ;
#4960=CARTESIAN_POINT ( 'NONE',  ( 114.0000000000000568, 64.53993994372673626, 18.52500000000035385 ) ) ;
#4968=AXIS2_PLACEMENT_3D ( 'NONE', #7352, #12147, #5916 ) ;
#4978=EDGE_LOOP ( 'NONE', ( #1147, #2629 ) ) ;
#4980=ORIENTED_EDGE ( 'NONE', *, *, #9956, .T. ) ;
#4984=VERTEX_POINT ( 'NONE', #10757 ) ;
#4988=ORIENTED_EDGE ( 'NONE', *, *, #7139, .F. ) ;
#4994=EDGE_CURVE ( 'NONE', #10303, #9977, #13493, .T. ) ;
#4997=VECTOR ( 'NONE', #11127, 1000.000000000000000 ) ;
#5000=ORIENTED_EDGE ( 'NONE', *, *, #6731, .F. ) ;
#5003=CIRCLE ( 'NONE', #10300, 3.525000000000000355 ) ;
#5007=DIRECTION ( 'NONE',  ( 0.000000000000000000, 0.000000000000000000, 1.000000000000000000 ) ) ;
#5008=EDGE_CURVE ( 'NONE', #9250, #14837, #7368, .T. ) ;
#5015=ORIENTED_EDGE ( 'NONE', *, *, #14306, .T. ) ;
#5016=CARTESIAN_POINT ( 'NONE',  ( 215.1062858801516882, 55.86394065090267702, 18.00000000000000355 ) ) ;
#5026=VECTOR ( 'NONE', #7066, 1000.000000000000000 ) ;
#5031=VECTOR ( 'NONE', #14387, 1000.000000000000000 ) ;
#5033=DIRECTION ( 'NONE',  ( 0.000000000000000000, 0.000000000000000000, 1.000000000000000000 ) ) ;
#5035=DIRECTION ( 'NONE',  ( -1.000000000000000000, 0.000000000000000000, 0.000000000000000000 ) ) ;
#5037=VERTEX_POINT ( 'NONE', #4913 ) ;
#5043=CIRCLE ( 'NONE', #2267, 1.499999999999994449 ) ;
#5046=CARTESIAN_POINT ( 'NONE',  ( -85.99999999999994316, 59.53993994372674337, 15.00000000000174794 ) ) ;
#5049=PLANE ( 'NONE',  #6144 ) ;
#5051=EDGE_CURVE ( 'NONE', #14374, #435, #5140, .T. ) ;
#5056=EDGE_LOOP ( 'NONE', ( #5767, #10997, #7932, #12354 ) ) ;
#5065=AXIS2_PLACEMENT_3D ( 'NONE', #350, #14657, #2908 ) ;
#5066=EDGE_CURVE ( 'NONE', #12693, #6470, #8701, .T. ) ;
#5071=LINE ( 'NONE', #81, #11098 ) ;
#5079=DIRECTION ( 'NONE',  ( -0.000000000000000000, 1.000000000000000000, -0.000000000000000000 ) ) ;
#5086=CARTESIAN_POINT ( 'NONE',  ( 164.0000000000000568, 64.53993994372673626, 13.29999999999999538 ) ) ;
#5093=CARTESIAN_POINT ( 'NONE',  ( 164.0000000000000568, 64.53993994372673626, 15.00000000000000355 ) ) ;
#5100=ORIENTED_EDGE ( 'NONE', *, *, #11840, .F. ) ;
#5108=VECTOR ( 'NONE', #931, 1000.000000000000000 ) ;
#5113=VERTEX_POINT ( 'NONE', #1495 ) ;
#5127=ORIENTED_EDGE ( 'NONE', *, *, #12744, .T. ) ;
#5131=DIRECTION ( 'NONE',  ( 0.000000000000000000, -1.000000000000000000, -1.156482317317871478E-16 ) ) ;
#5133=AXIS2_PLACEMENT_3D ( 'NONE', #4880, #11987, #4559 ) ;
#5140=LINE ( 'NONE', #9966, #2637 ) ;
#5141=CARTESIAN_POINT ( 'NONE',  ( 184.0000000000000568, 17.53993994372673271, 45.99999999999998579 ) ) ;
#5158=ORIENTED_EDGE ( 'NONE', *, *, #8786, .F. ) ;
#5159=FACE_OUTER_BOUND ( 'NONE', #4678, .T. ) ;
#5164=CARTESIAN_POINT ( 'NONE',  ( -63.50000000000002842, 17.53993994372674692, -17.50000000000002487 ) ) ;
#5167=DIRECTION ( 'NONE',  ( 0.000000000000000000, -0.000000000000000000, 1.000000000000000000 ) ) ;
#5190=CARTESIAN_POINT ( 'NONE',  ( -63.50000000000002842, 19.53993994372674692, -17.50000000000002487 ) ) ;
#5193=CARTESIAN_POINT ( 'NONE',  ( -63.50000000000002842, 19.53993994372673626, 52.49999999999997868 ) ) ;
#5196=DIRECTION ( 'NONE',  ( -0.000000000000000000, 1.000000000000000000, -0.000000000000000000 ) ) ;
#5198=CARTESIAN_POINT ( 'NONE',  ( 65.70000000000004547, 62.13993994372673768, 15.00000000000070166 ) ) ;
#5199=LINE ( 'NONE', #4003, #4199 ) ;
#5204=AXIS2_PLACEMENT_3D ( 'NONE', #4555, #9382, #4395 ) ;
#5209=VERTEX_POINT ( 'NONE', #5292 ) ;
#5211=ORIENTED_EDGE ( 'NONE', *, *, #6054, .F. ) ;
#5216=FACE_OUTER_BOUND ( 'NONE', #9265, .T. ) ;
#5232=ORIENTED_EDGE ( 'NONE', *, *, #8793, .T. ) ;
#5236=CYLINDRICAL_SURFACE ( 'NONE', #8989, 3.499999999999999556 ) ;
#5238=VECTOR ( 'NONE', #11587, 1000.000000000000000 ) ;
#5248=ORIENTED_EDGE ( 'NONE', *, *, #998, .F. ) ;
#5254=EDGE_CURVE ( 'NONE', #470, #11835, #11290, .T. ) ;
#5256=CARTESIAN_POINT ( 'NONE',  ( 184.0000000000000568, 19.53993994372674337, -12.49999999999999467 ) ) ;
#5258=DIRECTION ( 'NONE',  ( -0.000000000000000000, 1.000000000000000000, -0.000000000000000000 ) ) ;
#5261=LINE ( 'NONE', #9373, #2265 ) ;
#5263=LINE ( 'NONE', #5193, #12615 ) ;
#5267=DIRECTION ( 'NONE',  ( 0.000000000000000000, 0.000000000000000000, -1.000000000000000000 ) ) ;
#5269=LINE ( 'NONE', #2915, #7866 ) ;
#5271=DIRECTION ( 'NONE',  ( 0.000000000000000000, 0.000000000000000000, 1.000000000000000000 ) ) ;
#5274=EDGE_CURVE ( 'NONE', #9587, #5655, #11462, .T. ) ;
#5280=DIRECTION ( 'NONE',  ( -0.000000000000000000, 1.000000000000000000, -0.000000000000000000 ) ) ;
#5283=CARTESIAN_POINT ( 'NONE',  ( -70.00000000000000000, 19.53993994372673626, 48.99999999999997158 ) ) ;
#5290=DIRECTION ( 'NONE',  ( -0.000000000000000000, 1.000000000000000000, -0.000000000000000000 ) ) ;
#5292=CARTESIAN_POINT ( 'NONE',  ( -76.50000000000001421, 17.53993994372674692, -17.50000000000002487 ) ) ;
#5294=AXIS2_PLACEMENT_3D ( 'NONE', #2456, #8623, #13421 ) ;
#5295=CARTESIAN_POINT ( 'NONE',  ( -108.0000000000000568, 59.53993994372674337, 20.00000000000000355 ) ) ;
#5301=CARTESIAN_POINT ( 'NONE',  ( -85.99999999999994316, 59.53993994372674337, 16.70000000000174012 ) ) ;
#5303=DIRECTION ( 'NONE',  ( 0.000000000000000000, 0.000000000000000000, 1.000000000000000000 ) ) ;
#5308=DIRECTION ( 'NONE',  ( 0.000000000000000000, -1.486905836551548832E-16, 1.000000000000000000 ) ) ;
#5316=LINE ( 'NONE', #1327, #6981 ) ;
#5317=DIRECTION ( 'NONE',  ( -0.000000000000000000, 1.000000000000000000, -0.000000000000000000 ) ) ;
#5321=FACE_BOUND ( 'NONE', #15058, .T. ) ;
#5326=ADVANCED_FACE ( 'NONE', ( #5216 ), #8937, .T. ) ;
#5338=ORIENTED_EDGE ( 'NONE', *, *, #6815, .T. ) ;
#5340=CYLINDRICAL_SURFACE ( 'NONE', #94, 1.699999999999994849 ) ;
#5342=FACE_OUTER_BOUND ( 'NONE', #1738, .T. ) ;
#5352=DIRECTION ( 'NONE',  ( 0.000000000000000000, -1.000000000000000000, 0.000000000000000000 ) ) ;
#5354=DIRECTION ( 'NONE',  ( 0.000000000000000000, 0.000000000000000000, -1.000000000000000000 ) ) ;
#5357=CARTESIAN_POINT ( 'NONE',  ( 114.0000000000000568, 64.53993994372673626, 11.47500000000035136 ) ) ;
#5359=ORIENTED_EDGE ( 'NONE', *, *, #9809, .T. ) ;
#5360=DIRECTION ( 'NONE',  ( -1.000000000000000000, 0.000000000000000000, 0.000000000000000000 ) ) ;
#5361=CARTESIAN_POINT ( 'NONE',  ( -85.99999999999994316, 64.53993994372673626, 15.00000000000174794 ) ) ;
#5362=EDGE_CURVE ( 'NONE', #14837, #10092, #5759, .T. ) ;
#5368=EDGE_CURVE ( 'NONE', #5616, #973, #13677, .T. ) ;
#5370=EDGE_CURVE ( 'NONE', #9838, #3955, #9196, .T. ) ;
#5372=CARTESIAN_POINT ( 'NONE',  ( 14.00000000000004086, 59.53993994372674337, 15.00000000000104983 ) ) ;
#5375=DIRECTION ( 'NONE',  ( -0.000000000000000000, 1.000000000000000000, -0.000000000000000000 ) ) ;
#5380=ORIENTED_EDGE ( 'NONE', *, *, #10076, .F. ) ;
#5387=ADVANCED_FACE ( 'NONE', ( #5839 ), #1959, .F. ) ;
#5389=CARTESIAN_POINT ( 'NONE',  ( 164.0000000000000568, 59.53993994372674337, 15.00000000000000355 ) ) ;
#5399=PLANE ( 'NONE',  #737 ) ;
#5407=AXIS2_PLACEMENT_3D ( 'NONE', #1664, #5602, #15131 ) ;
#5410=ORIENTED_EDGE ( 'NONE', *, *, #346, .F. ) ;
#5414=ORIENTED_EDGE ( 'NONE', *, *, #1087, .T. ) ;
#5420=CARTESIAN_POINT ( 'NONE',  ( 195.1062858801516597, 40.86394065090267702, 16.00000000000001421 ) ) ;
#5425=DIRECTION ( 'NONE',  ( 0.000000000000000000, -1.486905836551548832E-16, 1.000000000000000000 ) ) ;
#5426=DIRECTION ( 'NONE',  ( -1.000000000000000000, -0.000000000000000000, -0.000000000000000000 ) ) ;
#5431=ORIENTED_EDGE ( 'NONE', *, *, #6089, .F. ) ;
#5439=AXIS2_PLACEMENT_3D ( 'NONE', #13349, #2551, #1427 ) ;
#5447=ORIENTED_EDGE ( 'NONE', *, *, #14332, .F. ) ;
#5451=FACE_OUTER_BOUND ( 'NONE', #8279, .T. ) ;
#5455=CARTESIAN_POINT ( 'NONE',  ( 114.0000000000000568, 64.51493994372674479, 15.00000000000035172 ) ) ;
#5456=AXIS2_PLACEMENT_3D ( 'NONE', #12720, #1910, #712 ) ;
#5457=EDGE_CURVE ( 'NONE', #14894, #9501, #851, .T. ) ;
#5466=DIRECTION ( 'NONE',  ( 0.000000000000000000, 0.000000000000000000, 1.000000000000000000 ) ) ;
#5468=AXIS2_PLACEMENT_3D ( 'NONE', #13477, #6315, #5271 ) ;
#5469=PLANE ( 'NONE',  #12491 ) ;
#5474=CARTESIAN_POINT ( 'NONE',  ( 114.0000000000000568, 64.51493994372674479, 11.50000000000034817 ) ) ;
#5478=DIRECTION ( 'NONE',  ( 0.000000000000000000, -1.000000000000000000, 0.000000000000000000 ) ) ;
#5480=CARTESIAN_POINT ( 'NONE',  ( -70.00000000000000000, 17.53993994372673271, 47.49999999999997868 ) ) ;
#5493=EDGE_CURVE ( 'NONE', #10896, #11184, #13429, .T. ) ;
#5498=DIRECTION ( 'NONE',  ( -0.000000000000000000, 1.000000000000000000, -0.000000000000000000 ) ) ;
#5504=VERTEX_POINT ( 'NONE', #1395 ) ;
#5507=EDGE_LOOP ( 'NONE', ( #6972, #11279, #14787, #7265 ) ) ;
#5519=CARTESIAN_POINT ( 'NONE',  ( -108.0000000000000568, 59.53993994372674337, 20.00000000000000355 ) ) ;
#5526=ORIENTED_EDGE ( 'NONE', *, *, #6341, .F. ) ;
#5528=VERTEX_POINT ( 'NONE', #1324 ) ;
#5531=PLANE ( 'NONE',  #12160 ) ;
#5537=ADVANCED_FACE ( 'NONE', ( #10817 ), #12068, .F. ) ;
#5539=ORIENTED_EDGE ( 'NONE', *, *, #11357, .T. ) ;
#5544=MANIFOLD_SOLID_BREP ( 'CBORE for M3 Pan Head Screw1[1]', #11667 ) ;
#5546=DIRECTION ( 'NONE',  ( -0.000000000000000000, 1.000000000000000000, -0.000000000000000000 ) ) ;
#5547=ORIENTED_EDGE ( 'NONE', *, *, #12429, .F. ) ;
#5554=VECTOR ( 'NONE', #5896, 1000.000000000000114 ) ;
#5566=CARTESIAN_POINT ( 'NONE',  ( 177.5000000000000853, 17.53993994372674692, -17.50000000000002487 ) ) ;
#5572=EDGE_CURVE ( 'NONE', #13310, #5662, #8177, .T. ) ;
#5573=EDGE_CURVE ( 'NONE', #6899, #2171, #8995, .T. ) ;
#5574=EDGE_CURVE ( 'NONE', #6095, #11949, #356, .T. ) ;
#5575=LINE ( 'NONE', #2160, #979 ) ;
#5578=CARTESIAN_POINT ( 'NONE',  ( 64.00000000000005684, 64.53993994372673626, 15.00000000000070166 ) ) ;
#5585=DIRECTION ( 'NONE',  ( 0.000000000000000000, 0.000000000000000000, 1.000000000000000000 ) ) ;
#5586=CARTESIAN_POINT ( 'NONE',  ( 164.0000000000000568, 64.53993994372673626, 15.00000000000000355 ) ) ;
#5590=VERTEX_POINT ( 'NONE', #11353 ) ;
#5593=CARTESIAN_POINT ( 'NONE',  ( 114.0000000000000568, 59.53993994372674337, 13.30000000000035776 ) ) ;
#5594=DIRECTION ( 'NONE',  ( 0.000000000000000000, 0.000000000000000000, 1.000000000000000000 ) ) ;
#5595=LINE ( 'NONE', #10405, #2365 ) ;
#5599=AXIS2_PLACEMENT_3D ( 'NONE', #2358, #11995, #7112 ) ;
#5602=DIRECTION ( 'NONE',  ( 0.000000000000000000, 8.673617379884035472E-17, -1.000000000000000000 ) ) ;
#5605=ORIENTED_EDGE ( 'NONE', *, *, #12118, .F. ) ;
#5612=FACE_OUTER_BOUND ( 'NONE', #4978, .T. ) ;
#5615=EDGE_CURVE ( 'NONE', #15409, #973, #14807, .T. ) ;
#5616=VERTEX_POINT ( 'NONE', #598 ) ;
#5632=AXIS2_PLACEMENT_3D ( 'NONE', #13787, #2985, #6471 ) ;
#5644=VECTOR ( 'NONE', #14793, 1000.000000000000000 ) ;
#5647=PLANE ( 'NONE',  #7820 ) ;
#5649=APPLICATION_CONTEXT ( 'automotive_design' ) ;
#5650=EDGE_CURVE ( 'NONE', #9401, #9986, #4002, .T. ) ;
#5651=DIRECTION ( 'NONE',  ( -0.000000000000000000, 1.000000000000000000, -0.000000000000000000 ) ) ;
#5654=EDGE_CURVE ( 'NONE', #10742, #627, #1560, .T. ) ;
#5655=VERTEX_POINT ( 'NONE', #13631 ) ;
#5661=FACE_OUTER_BOUND ( 'NONE', #8705, .T. ) ;
#5662=VERTEX_POINT ( 'NONE', #12758 ) ;
#5665=EDGE_LOOP ( 'NONE', ( #12551, #11141, #6260, #14386 ) ) ;
#5666=CARTESIAN_POINT ( 'NONE',  ( -35.99999999999995026, 64.51493994372674479, 18.50000000000140332 ) ) ;
#5667=LINE ( 'NONE', #2986, #12297 ) ;
#5668=VECTOR ( 'NONE', #10045, 1000.000000000000000 ) ;
#5681=DIRECTION ( 'NONE',  ( 1.000000000000000000, 0.000000000000000000, 0.000000000000000000 ) ) ;
#5684=LINE ( 'NONE', #15287, #7624 ) ;
#5685=ORIENTED_EDGE ( 'NONE', *, *, #1988, .T. ) ;
#5687=LINE ( 'NONE', #10268, #8115 ) ;
#5688=ADVANCED_FACE ( 'NONE', ( #4468 ), #6862, .F. ) ;
#5689=VECTOR ( 'NONE', #13268, 1000.000000000000000 ) ;
#5702=CARTESIAN_POINT ( 'NONE',  ( -85.99999999999994316, 59.53993994372674337, 16.70000000000174012 ) ) ;
#5707=EDGE_CURVE ( 'NONE', #11511, #14374, #990, .T. ) ;
#5711=AXIS2_PLACEMENT_3D ( 'NONE', #13301, #1076, #14412 ) ;
#5720=VERTEX_POINT ( 'NONE', #15123 ) ;
#5734=PLANE ( 'NONE',  #13325 ) ;
#5737=ORIENTED_EDGE ( 'NONE', *, *, #14334, .F. ) ;
#5740=FACE_BOUND ( 'NONE', #14156, .T. ) ;
#5745=CIRCLE ( 'NONE', #8031, 3.525000000000002132 ) ;
#5752=LINE ( 'NONE', #15597, #1057 ) ;
#5754=AXIS2_PLACEMENT_3D ( 'NONE', #1933, #13702, #5585 ) ;
#5759=LINE ( 'NONE', #6957, #2605 ) ;
#5762=VECTOR ( 'NONE', #4188, 1000.000000000000000 ) ;
#5767=ORIENTED_EDGE ( 'NONE', *, *, #3700, .F. ) ;
#5769=CARTESIAN_POINT ( 'NONE',  ( -35.99999999999995026, 64.53993994372673626, 16.70000000000140261 ) ) ;
#5775=DIRECTION ( 'NONE',  ( 0.000000000000000000, -1.000000000000000000, 0.000000000000000000 ) ) ;
#5776=CIRCLE ( 'NONE', #7812, 3.525000000000002132 ) ;
#5778=CARTESIAN_POINT ( 'NONE',  ( -35.99999999999995026, 64.51493994372674479, 15.00000000000139977 ) ) ;
#5786=ADVANCED_FACE ( 'NONE', ( #8135 ), #1075, .F. ) ;
#5792=UNCERTAINTY_MEASURE_WITH_UNIT (LENGTH_MEASURE( 1.000000000000000082E-05 ), #5834, 'distance_accuracy_value', 'NONE');
#5801=VECTOR ( 'NONE', #15237, 1000.000000000000000 ) ;
#5803=CIRCLE ( 'NONE', #14620, 1.699999999999996625 ) ;
#5812=CARTESIAN_POINT ( 'NONE',  ( -110.0000000000000426, 59.53993994372674337, 10.00000000000000178 ) ) ;
#5817=DIRECTION ( 'NONE',  ( 0.000000000000000000, -0.000000000000000000, -1.000000000000000000 ) ) ;
#5828=EDGE_CURVE ( 'NONE', #12024, #6168, #3614, .T. ) ;
#5829=DIRECTION ( 'NONE',  ( 0.000000000000000000, 0.000000000000000000, 1.000000000000000000 ) ) ;
#5834=( LENGTH_UNIT ( ) NAMED_UNIT ( * ) SI_UNIT ( .MILLI., .METRE. ) );
#5836=DIRECTION ( 'NONE',  ( -0.000000000000000000, 1.000000000000000000, -0.000000000000000000 ) ) ;
#5839=FACE_OUTER_BOUND ( 'NONE', #11199, .T. ) ;
#5843=EDGE_CURVE ( 'NONE', #11923, #6265, #5595, .T. ) ;
#5849=ADVANCED_FACE ( 'NONE', ( #10799 ), #12438, .F. ) ;
#5855=ORIENTED_EDGE ( 'NONE', *, *, #4899, .T. ) ;
#5857=ORIENTED_EDGE ( 'NONE', *, *, #9134, .T. ) ;
#5860=CARTESIAN_POINT ( 'NONE',  ( -110.0000000000000426, 19.53993994372674337, 9.999999999999998224 ) ) ;
#5861=ORIENTED_EDGE ( 'NONE', *, *, #10392, .T. ) ;
#5863=DIRECTION ( 'NONE',  ( -0.000000000000000000, 1.000000000000000000, -0.000000000000000000 ) ) ;
#5866=AXIS2_PLACEMENT_3D ( 'NONE', #7656, #7577, #4085 ) ;
#5870=EDGE_CURVE ( 'NONE', #2296, #13310, #2346, .T. ) ;
#5877=ORIENTED_EDGE ( 'NONE', *, *, #7094, .F. ) ;
#5884=EDGE_LOOP ( 'NONE', ( #1110, #2395 ) ) ;
#5890=FACE_BOUND ( 'NONE', #659, .T. ) ;
#5893=ORIENTED_EDGE ( 'NONE', *, *, #5574, .F. ) ;
#5896=DIRECTION ( 'NONE',  ( 8.659560562354932858E-17, 0.7071067811865474617, -0.7071067811865474617 ) ) ;
#5901=VECTOR ( 'NONE', #13304, 1000.000000000000000 ) ;
#5904=CARTESIAN_POINT ( 'NONE',  ( 200.1062858801516597, 40.86394065090267702, -219.0000000000000853 ) ) ;
#5909=DIRECTION ( 'NONE',  ( 0.000000000000000000, -1.000000000000000000, 0.000000000000000000 ) ) ;
#5910=ORIENTED_EDGE ( 'NONE', *, *, #2719, .F. ) ;
#5915=DIRECTION ( 'NONE',  ( 0.000000000000000000, 0.000000000000000000, 1.000000000000000000 ) ) ;
#5916=DIRECTION ( 'NONE',  ( 0.000000000000000000, -0.000000000000000000, -1.000000000000000000 ) ) ;
#5919=VECTOR ( 'NONE', #2903, 1000.000000000000000 ) ;
#5925=ORIENTED_EDGE ( 'NONE', *, *, #13174, .T. ) ;
#5926=EDGE_LOOP ( 'NONE', ( #8509, #3786, #3498, #221 ) ) ;
#5927=CARTESIAN_POINT ( 'NONE',  ( -85.99999999999994316, 56.53993994372675047, 15.00000000000174794 ) ) ;
#5932=DIRECTION ( 'NONE',  ( 0.000000000000000000, 0.000000000000000000, -1.000000000000000000 ) ) ;
#5937=VERTEX_POINT ( 'NONE', #3680 ) ;
#5938=PRESENTATION_STYLE_ASSIGNMENT (( #11789 ) ) ;
#5941=ORIENTED_EDGE ( 'NONE', *, *, #13549, .F. ) ;
#5946=ORIENTED_EDGE ( 'NONE', *, *, #3398, .F. ) ;
#5947=VERTEX_POINT ( 'NONE', #8589 ) ;
#5951=VERTEX_POINT ( 'NONE', #178 ) ;
#5974=ORIENTED_EDGE ( 'NONE', *, *, #8029, .F. ) ;
#5978=DIRECTION ( 'NONE',  ( -0.000000000000000000, 1.000000000000000000, -0.000000000000000000 ) ) ;
#5982=PLANE ( 'NONE',  #3871 ) ;
#5992=ORIENTED_EDGE ( 'NONE', *, *, #14994, .F. ) ;
#5993=DIRECTION ( 'NONE',  ( 0.000000000000000000, 0.000000000000000000, -1.000000000000000000 ) ) ;
#5996=PRESENTATION_STYLE_ASSIGNMENT (( #1166 ) ) ;
#6000=EDGE_LOOP ( 'NONE', ( #7284, #5380 ) ) ;
#6009=ORIENTED_EDGE ( 'NONE', *, *, #3398, .T. ) ;
#6013=EDGE_LOOP ( 'NONE', ( #11794, #3789 ) ) ;
#6018=CARTESIAN_POINT ( 'NONE',  ( 14.00000000000004086, 56.53993994372675047, 15.00000000000104983 ) ) ;
#6020=ORIENTED_EDGE ( 'NONE', *, *, #59, .F. ) ;
#6026=CARTESIAN_POINT ( 'NONE',  ( -85.99999999999994316, 64.53993994372673626, 16.70000000000174012 ) ) ;
#6029=DIRECTION ( 'NONE',  ( -0.000000000000000000, 1.000000000000000000, -0.000000000000000000 ) ) ;
#6035=ORIENTED_EDGE ( 'NONE', *, *, #422, .T. ) ;
#6051=AXIS2_PLACEMENT_3D ( 'NONE', #6746, #6822, #10737 ) ;
#6054=EDGE_CURVE ( 'NONE', #5655, #9587, #80, .T. ) ;
#6055=VERTEX_POINT ( 'NONE', #14789 ) ;
#6060=ORIENTED_EDGE ( 'NONE', *, *, #11252, .F. ) ;
#6067=VECTOR ( 'NONE', #12999, 1000.000000000000000 ) ;
#6073=CARTESIAN_POINT ( 'NONE',  ( 14.00000000000004086, 64.53993994372673626, 13.30000000000105231 ) ) ;
#6075=CIRCLE ( 'NONE', #11864, 3.500000000000004885 ) ;
#6078=AXIS2_PLACEMENT_3D ( 'NONE', #6892, #14283, #3692 ) ;
#6080=CARTESIAN_POINT ( 'NONE',  ( 64.00000000000005684, 64.53993994372673626, 18.50000000000070344 ) ) ;
#6083=SURFACE_STYLE_FILL_AREA ( #7199 ) ;
#6089=EDGE_CURVE ( 'NONE', #8626, #6095, #6291, .T. ) ;
#6095=VERTEX_POINT ( 'NONE', #11260 ) ;
#6096=DIRECTION ( 'NONE',  ( -0.000000000000000000, 1.000000000000000000, -0.000000000000000000 ) ) ;
#6106=DIRECTION ( 'NONE',  ( -0.000000000000000000, 1.000000000000000000, -0.000000000000000000 ) ) ;
#6107=CIRCLE ( 'NONE', #13649, 1.499999999999997780 ) ;
#6108=EDGE_LOOP ( 'NONE', ( #13341, #782, #1902, #5359 ) ) ;
#6111=ORIENTED_EDGE ( 'NONE', *, *, #13657, .F. ) ;
#6112=ORIENTED_EDGE ( 'NONE', *, *, #2051, .F. ) ;
#6115=ORIENTED_EDGE ( 'NONE', *, *, #6986, .T. ) ;
#6116=AXIS2_PLACEMENT_3D ( 'NONE', #8572, #3745, #2483 ) ;
#6121=VERTEX_POINT ( 'NONE', #1773 ) ;
#6125=ORIENTED_EDGE ( 'NONE', *, *, #11584, .T. ) ;
#6129=DIRECTION ( 'NONE',  ( 0.000000000000000000, 1.000000000000000000, 1.156482317317871725E-16 ) ) ;
#6133=LINE ( 'NONE', #7249, #9363 ) ;
#6137=DIRECTION ( 'NONE',  ( -0.000000000000000000, 1.000000000000000000, -0.000000000000000000 ) ) ;
#6139=CARTESIAN_POINT ( 'NONE',  ( -85.99999999999994316, 64.53993994372673626, 15.00000000000174794 ) ) ;
#6140=DIRECTION ( 'NONE',  ( -0.000000000000000000, 1.000000000000000000, -0.000000000000000000 ) ) ;
#6142=EDGE_CURVE ( 'NONE', #10019, #8250, #4635, .T. ) ;
#6144=AXIS2_PLACEMENT_3D ( 'NONE', #13408, #7505, #11052 ) ;
#6146=EDGE_CURVE ( 'NONE', #3552, #6055, #7939, .T. ) ;
#6147=FACE_OUTER_BOUND ( 'NONE', #6961, .T. ) ;
#6157=AXIS2_PLACEMENT_3D ( 'NONE', #5361, #5280, #6787 ) ;
#6160=DIRECTION ( 'NONE',  ( 0.000000000000000000, 0.000000000000000000, -1.000000000000000000 ) ) ;
#6161=CARTESIAN_POINT ( 'NONE',  ( -70.00000000000000000, 17.53993994372673271, 45.99999999999998579 ) ) ;
#6168=VERTEX_POINT ( 'NONE', #10465 ) ;
#6176=LINE ( 'NONE', #139, #11317 ) ;
#6178=ADVANCED_FACE ( 'NONE', ( #9132 ), #6918, .T. ) ;
#6181=DIRECTION ( 'NONE',  ( -0.000000000000000000, 1.486905836551548832E-16, -1.000000000000000000 ) ) ;
#6182=AXIS2_PLACEMENT_3D ( 'NONE', #14794, #5258, #5033 ) ;
#6183=CARTESIAN_POINT ( 'NONE',  ( 164.0000000000000568, 64.53993994372673626, 15.00000000000000355 ) ) ;
#6186=DIRECTION ( 'NONE',  ( -0.000000000000000000, 1.000000000000000000, -0.000000000000000000 ) ) ;
#6189=CIRCLE ( 'NONE', #7452, 3.525000000000002132 ) ;
#6192=ORIENTED_EDGE ( 'NONE', *, *, #2262, .F. ) ;
#6193=VERTEX_POINT ( 'NONE', #2086 ) ;
#6201=ORIENTED_EDGE ( 'NONE', *, *, #5573, .F. ) ;
#6205=ORIENTED_EDGE ( 'NONE', *, *, #8793, .F. ) ;
#6207=DIRECTION ( 'NONE',  ( -0.000000000000000000, 1.000000000000000000, -0.000000000000000000 ) ) ;
#6213=VECTOR ( 'NONE', #8240, 1000.000000000000000 ) ;
#6215=ORIENTED_EDGE ( 'NONE', *, *, #998, .T. ) ;
#6218=EDGE_CURVE ( 'NONE', #1700, #6193, #12662, .T. ) ;
#6221=DIRECTION ( 'NONE',  ( 0.000000000000000000, 0.000000000000000000, 1.000000000000000000 ) ) ;
#6225=CARTESIAN_POINT ( 'NONE',  ( -35.99999999999995026, 64.51493994372674479, 15.00000000000139977 ) ) ;
#6230=CARTESIAN_POINT ( 'NONE',  ( 177.5000000000000853, 17.53993994372674692, -17.50000000000002487 ) ) ;
#6231=DIRECTION ( 'NONE',  ( -0.000000000000000000, -0.000000000000000000, 1.000000000000000000 ) ) ;
#6238=DIRECTION ( 'NONE',  ( 0.000000000000000000, 0.000000000000000000, 1.000000000000000000 ) ) ;
#6245=ADVANCED_FACE ( 'NONE', ( #6759 ), #5647, .F. ) ;
#6247=ORIENTED_EDGE ( 'NONE', *, *, #15415, .F. ) ;
#6259=DIRECTION ( 'NONE',  ( 1.000000000000000000, 0.000000000000000000, 0.000000000000000000 ) ) ;
#6260=ORIENTED_EDGE ( 'NONE', *, *, #14994, .T. ) ;
#6265=VERTEX_POINT ( 'NONE', #3355 ) ;
#6277=EDGE_CURVE ( 'NONE', #15478, #1467, #5575, .T. ) ;
#6281=DIRECTION ( 'NONE',  ( -0.000000000000000000, -0.000000000000000000, -1.000000000000000000 ) ) ;
#6284=CARTESIAN_POINT ( 'NONE',  ( -85.99999999999994316, 64.53993994372673626, 18.52500000000175007 ) ) ;
#6290=AXIS2_PLACEMENT_3D ( 'NONE', #5389, #13820, #1512 ) ;
#6291=LINE ( 'NONE', #4138, #13970 ) ;
#6295=LINE ( 'NONE', #3918, #5644 ) ;
#6300=DIRECTION ( 'NONE',  ( 0.000000000000000000, 0.000000000000000000, 1.000000000000000000 ) ) ;
#6302=ORIENTED_EDGE ( 'NONE', *, *, #14370, .F. ) ;
#6307=AXIS2_PLACEMENT_3D ( 'NONE', #910, #8512, #6939 ) ;
#6309=CARTESIAN_POINT ( 'NONE',  ( -63.50000000000002842, 17.53993994372673271, 52.49999999999997868 ) ) ;
#6310=CARTESIAN_POINT ( 'NONE',  ( 215.1062858801516882, 25.86394065090268057, 13.00000000000000178 ) ) ;
#6311=AXIS2_PLACEMENT_3D ( 'NONE', #2073, #11717, #4518 ) ;
#6313=VECTOR ( 'NONE', #711, 1000.000000000000000 ) ;
#6314=DIRECTION ( 'NONE',  ( 0.000000000000000000, 0.000000000000000000, 1.000000000000000000 ) ) ;
#6315=DIRECTION ( 'NONE',  ( -0.000000000000000000, 1.000000000000000000, -0.000000000000000000 ) ) ;
#6317=CARTESIAN_POINT ( 'NONE',  ( -108.0000000000000568, 59.53993994372674337, 20.00000000000000355 ) ) ;
#6330=DIRECTION ( 'NONE',  ( 0.000000000000000000, 0.000000000000000000, 1.000000000000000000 ) ) ;
#6335=AXIS2_PLACEMENT_3D ( 'NONE', #11765, #14196, #3395 ) ;
#6337=CIRCLE ( 'NONE', #7856, 1.699999999999991518 ) ;
#6341=EDGE_CURVE ( 'NONE', #12779, #15030, #10859, .T. ) ;
#6348=CIRCLE ( 'NONE', #15142, 3.500000000000004885 ) ;
#6353=CARTESIAN_POINT ( 'NONE',  ( 14.00000000000004086, 64.53993994372673626, 16.70000000000104734 ) ) ;
#6355=EDGE_LOOP ( 'NONE', ( #9140, #3585 ) ) ;
#6358=LINE ( 'NONE', #14776, #9848 ) ;
#6362=FACE_BOUND ( 'NONE', #3522, .T. ) ;
#6365=PLANE ( 'NONE',  #10373 ) ;
#6378=CARTESIAN_POINT ( 'NONE',  ( 164.0000000000000568, 59.53993994372674337, 15.00000000000000355 ) ) ;
#6386=CARTESIAN_POINT ( 'NONE',  ( 164.0000000000000568, 59.53993994372674337, 15.00000000000000355 ) ) ;
#6393=LINE ( 'NONE', #9944, #7778 ) ;
#6394=DIRECTION ( 'NONE',  ( 0.000000000000000000, 0.000000000000000000, 1.000000000000000000 ) ) ;
#6395=DIRECTION ( 'NONE',  ( -0.000000000000000000, 1.000000000000000000, -0.000000000000000000 ) ) ;
#6401=ORIENTED_EDGE ( 'NONE', *, *, #14847, .T. ) ;
#6406=ORIENTED_EDGE ( 'NONE', *, *, #9109, .T. ) ;
#6409=ORIENTED_EDGE ( 'NONE', *, *, #10977, .F. ) ;
#6411=CARTESIAN_POINT ( 'NONE',  ( 224.0000000000000853, 19.53993994372674337, 24.99999999999999645 ) ) ;
#6414=DIRECTION ( 'NONE',  ( -0.000000000000000000, -0.000000000000000000, 1.000000000000000000 ) ) ;
#6416=DIRECTION ( 'NONE',  ( 0.000000000000000000, -1.000000000000000000, 0.000000000000000000 ) ) ;
#6418=ADVANCED_BREP_SHAPE_REPRESENTATION ( '', ( #5544, #11070, #12337 ), #4262 ) ;
#6423=CARTESIAN_POINT ( 'NONE',  ( 194.0000000000000568, 59.53993994372674337, 10.00000000000000178 ) ) ;
#6433=EDGE_CURVE ( 'NONE', #13079, #9297, #11959, .T. ) ;
#6435=CARTESIAN_POINT ( 'NONE',  ( -110.0000000000000426, 59.53993994372674337, 25.00000000000000000 ) ) ;
#6441=DIRECTION ( 'NONE',  ( -0.000000000000000000, 1.000000000000000000, -0.000000000000000000 ) ) ;
#6455=DIRECTION ( 'NONE',  ( 0.000000000000000000, -1.000000000000000000, 0.000000000000000000 ) ) ;
#6470=VERTEX_POINT ( 'NONE', #2877 ) ;
#6471=DIRECTION ( 'NONE',  ( 0.000000000000000000, 0.000000000000000000, 1.000000000000000000 ) ) ;
#6477=ORIENTED_EDGE ( 'NONE', *, *, #3272, .F. ) ;
#6484=ADVANCED_FACE ( 'NONE', ( #12255 ), #9987, .F. ) ;
#6491=DIRECTION ( 'NONE',  ( 0.000000000000000000, -0.000000000000000000, -1.000000000000000000 ) ) ;
#6492=ORIENTED_EDGE ( 'NONE', *, *, #2623, .F. ) ;
#6499=EDGE_LOOP ( 'NONE', ( #349, #4720, #13528, #8243 ) ) ;
#6500=CARTESIAN_POINT ( 'NONE',  ( -35.99999999999995026, 64.53993994372673626, 18.50000000000140332 ) ) ;
#6503=DIRECTION ( 'NONE',  ( 0.000000000000000000, 0.7071067811865474617, 0.7071067811865474617 ) ) ;
#6511=CARTESIAN_POINT ( 'NONE',  ( -110.0000000000000426, 19.53993994372674337, 24.99999999999999645 ) ) ;
#6515=CARTESIAN_POINT ( 'NONE',  ( 164.0000000000000568, 59.53993994372674337, 13.29999999999999538 ) ) ;
#6537=DIRECTION ( 'NONE',  ( -0.000000000000000000, 1.000000000000000000, -0.000000000000000000 ) ) ;
#6539=LINE ( 'NONE', #7564, #15480 ) ;
#6541=LINE ( 'NONE', #7887, #14815 ) ;
#6542=VECTOR ( 'NONE', #1164, 1000.000000000000000 ) ;
#6545=ORIENTED_EDGE ( 'NONE', *, *, #11057, .T. ) ;
#6548=EDGE_LOOP ( 'NONE', ( #10917, #13473, #3091, #4371 ) ) ;
#6559=DIRECTION ( 'NONE',  ( 0.000000000000000000, 0.000000000000000000, 1.000000000000000000 ) ) ;
#6561=AXIS2_PLACEMENT_3D ( 'NONE', #10631, #11893, #10709 ) ;
#6563=ORIENTED_EDGE ( 'NONE', *, *, #7244, .T. ) ;
#6565=ADVANCED_FACE ( 'NONE', ( #321, #5159 ), #5399, .F. ) ;
#6573=DIRECTION ( 'NONE',  ( 0.000000000000000000, 0.000000000000000000, 1.000000000000000000 ) ) ;
#6587=AXIS2_PLACEMENT_3D ( 'NONE', #13570, #11529, #10347 ) ;
#6589=VERTEX_POINT ( 'NONE', #11546 ) ;
#6594=DIRECTION ( 'NONE',  ( -0.000000000000000000, 1.000000000000000000, 1.156482317317871725E-16 ) ) ;
#6601=VERTEX_POINT ( 'NONE', #1909 ) ;
#6607=VERTEX_POINT ( 'NONE', #1833 ) ;
#6610=EDGE_CURVE ( 'NONE', #8626, #4614, #9551, .T. ) ;
#6617=DIRECTION ( 'NONE',  ( 0.000000000000000000, 0.000000000000000000, -1.000000000000000000 ) ) ;
#6619=CIRCLE ( 'NONE', #2054, 3.499999999999999556 ) ;
#6622=FACE_OUTER_BOUND ( 'NONE', #4735, .T. ) ;
#6625=ORIENTED_EDGE ( 'NONE', *, *, #9348, .F. ) ;
#6642=FACE_OUTER_BOUND ( 'NONE', #1930, .T. ) ;
#6645=ORIENTED_EDGE ( 'NONE', *, *, #12136, .T. ) ;
#6650=EDGE_CURVE ( 'NONE', #11835, #15158, #3779, .T. ) ;
#6656=AXIS2_PLACEMENT_3D ( 'NONE', #13318, #9712, #14426 ) ;
#6658=ORIENTED_EDGE ( 'NONE', *, *, #3215, .T. ) ;
#6664=LINE ( 'NONE', #13817, #629 ) ;
#6669=ORIENTED_EDGE ( 'NONE', *, *, #10791, .T. ) ;
#6673=CARTESIAN_POINT ( 'NONE',  ( 15.70000000000004015, 62.13993994372673768, 15.00000000000104983 ) ) ;
#6683=TOROIDAL_SURFACE ( 'NONE', #5407, 6.999999999999991118, 2.000000000000000000 ) ;
#6692=CYLINDRICAL_SURFACE ( 'NONE', #12862, 1.699999999999993072 ) ;
#6693=CIRCLE ( 'NONE', #3147, 1.499999999999994449 ) ;
#6702=ORIENTED_EDGE ( 'NONE', *, *, #4517, .T. ) ;
#6704=VECTOR ( 'NONE', #2960, 1000.000000000000000 ) ;
#6708=CARTESIAN_POINT ( 'NONE',  ( 14.00000000000004086, 64.53993994372673626, 11.47500000000104947 ) ) ;
#6709=ADVANCED_FACE ( 'NONE', ( #11479 ), #2782, .F. ) ;
#6716=VECTOR ( 'NONE', #2325, 1000.000000000000000 ) ;
#6727=CIRCLE ( 'NONE', #5204, 3.500000000000004885 ) ;
#6731=EDGE_CURVE ( 'NONE', #2171, #868, #5043, .T. ) ;
#6733=ADVANCED_FACE ( 'NONE', ( #10902 ), #9714, .T. ) ;
#6736=AXIS2_PLACEMENT_3D ( 'NONE', #8685, #10024, #2917 ) ;
#6742=CARTESIAN_POINT ( 'NONE',  ( -63.50000000000002842, 19.53993994372674692, -17.50000000000002487 ) ) ;
#6746=CARTESIAN_POINT ( 'NONE',  ( 207.1062858801516597, 40.86394065090267702, 16.00000000000001421 ) ) ;
#6747=CARTESIAN_POINT ( 'NONE',  ( -35.99999999999995026, 64.53993994372673626, 15.00000000000139977 ) ) ;
#6748=CARTESIAN_POINT ( 'NONE',  ( 64.00000000000005684, 64.53993994372673626, 15.00000000000070166 ) ) ;
#6749=DIRECTION ( 'NONE',  ( 1.000000000000000000, -0.000000000000000000, -0.000000000000000000 ) ) ;
#6750=EDGE_LOOP ( 'NONE', ( #8470, #13640, #14801, #4601 ) ) ;
#6753=PLANE ( 'NONE',  #1745 ) ;
#6759=FACE_OUTER_BOUND ( 'NONE', #3736, .T. ) ;
#6766=ORIENTED_EDGE ( 'NONE', *, *, #9676, .T. ) ;
#6767=FACE_OUTER_BOUND ( 'NONE', #6108, .T. ) ;
#6775=EDGE_LOOP ( 'NONE', ( #3171, #3472 ) ) ;
#6777=DIRECTION ( 'NONE',  ( 0.000000000000000000, -1.000000000000000000, -1.156482317317871478E-16 ) ) ;
#6781=EDGE_CURVE ( 'NONE', #61, #12693, #11047, .T. ) ;
#6787=DIRECTION ( 'NONE',  ( 0.000000000000000000, 0.000000000000000000, 1.000000000000000000 ) ) ;
#6805=VERTEX_POINT ( 'NONE', #3626 ) ;
#6809=ORIENTED_EDGE ( 'NONE', *, *, #11499, .F. ) ;
#6815=EDGE_CURVE ( 'NONE', #3946, #649, #11337, .T. ) ;
#6820=AXIS2_PLACEMENT_3D ( 'NONE', #3373, #8441, #4628 ) ;
#6822=DIRECTION ( 'NONE',  ( -1.224646799147353207E-16, 1.000000000000000000, 0.000000000000000000 ) ) ;
#6830=DIRECTION ( 'NONE',  ( -0.000000000000000000, 1.000000000000000000, -0.000000000000000000 ) ) ;
#6833=AXIS2_PLACEMENT_3D ( 'NONE', #181, #4953, #7335 ) ;
#6838=ORIENTED_EDGE ( 'NONE', *, *, #2084, .F. ) ;
#6840=DIRECTION ( 'NONE',  ( 0.000000000000000000, 0.000000000000000000, -1.000000000000000000 ) ) ;
#6841=CARTESIAN_POINT ( 'NONE',  ( -85.99999999999994316, 64.51493994372674479, 15.00000000000174794 ) ) ;
#6845=VECTOR ( 'NONE', #2101, 1000.000000000000000 ) ;
#6850=CARTESIAN_POINT ( 'NONE',  ( -63.50000000000002842, 19.53993994372673626, 52.49999999999997868 ) ) ;
#6859=VECTOR ( 'NONE', #6281, 1000.000000000000000 ) ;
#6860=LINE ( 'NONE', #11671, #12359 ) ;
#6862=CYLINDRICAL_SURFACE ( 'NONE', #6905, 3.500000000000004885 ) ;
#6867=DIRECTION ( 'NONE',  ( 0.000000000000000000, -1.000000000000000000, -1.156482317317871478E-16 ) ) ;
#6871=CARTESIAN_POINT ( 'NONE',  ( -76.50000000000001421, 19.53993994372674692, -17.50000000000002487 ) ) ;
#6872=ADVANCED_FACE ( 'NONE', ( #13404 ), #14431, .F. ) ;
#6892=CARTESIAN_POINT ( 'NONE',  ( 164.0000000000000568, 64.53993994372673626, 15.00000000000000355 ) ) ;
#6899=VERTEX_POINT ( 'NONE', #6161 ) ;
#6900=LINE ( 'NONE', #4355, #8344 ) ;
#6901=EDGE_CURVE ( 'NONE', #9730, #163, #13321, .T. ) ;
#6903=CARTESIAN_POINT ( 'NONE',  ( 200.1062858801516597, 40.86394065090267702, -219.0000000000000853 ) ) ;
#6905=AXIS2_PLACEMENT_3D ( 'NONE', #12920, #15350, #2107 ) ;
#6907=FACE_OUTER_BOUND ( 'NONE', #6963, .T. ) ;
#6911=ORIENTED_EDGE ( 'NONE', *, *, #3852, .F. ) ;
#6918=PLANE ( 'NONE',  #8325 ) ;
#6925=CYLINDRICAL_SURFACE ( 'NONE', #8896, 1.699999999999993072 ) ;
#6926=ORIENTED_EDGE ( 'NONE', *, *, #5362, .T. ) ;
#6934=DIRECTION ( 'NONE',  ( -0.000000000000000000, 1.000000000000000000, -0.000000000000000000 ) ) ;
#6935=CARTESIAN_POINT ( 'NONE',  ( 164.0000000000000568, 64.53993994372673626, 15.00000000000000355 ) ) ;
#6937=ORIENTED_EDGE ( 'NONE', *, *, #14626, .T. ) ;
#6939=DIRECTION ( 'NONE',  ( 0.000000000000000000, 0.000000000000000000, 1.000000000000000000 ) ) ;
#6941=DIRECTION ( 'NONE',  ( 0.000000000000000000, 0.000000000000000000, 1.000000000000000000 ) ) ;
#6951=FACE_OUTER_BOUND ( 'NONE', #12778, .T. ) ;
#6957=CARTESIAN_POINT ( 'NONE',  ( 177.5000000000000853, 19.53993994372673626, 52.49999999999997868 ) ) ;
#6961=EDGE_LOOP ( 'NONE', ( #15371, #8235, #4871, #7713 ) ) ;
#6963=EDGE_LOOP ( 'NONE', ( #4186, #13539, #8005, #15456 ) ) ;
#6967=DIRECTION ( 'NONE',  ( -0.000000000000000000, 1.000000000000000000, -0.000000000000000000 ) ) ;
#6972=ORIENTED_EDGE ( 'NONE', *, *, #7180, .T. ) ;
#6981=VECTOR ( 'NONE', #2442, 1000.000000000000000 ) ;
#6984=SURFACE_SIDE_STYLE ('',( #8327 ) ) ;
#6986=EDGE_CURVE ( 'NONE', #4984, #12099, #15122, .T. ) ;
#6994=DIRECTION ( 'NONE',  ( 1.000000000000000000, 0.000000000000000000, 0.000000000000000000 ) ) ;
#6996=DIRECTION ( 'NONE',  ( 0.000000000000000000, -1.000000000000000000, 0.000000000000000000 ) ) ;
#7000=AXIS2_PLACEMENT_3D ( 'NONE', #4087, #8919, #5354 ) ;
#7002=DIRECTION ( 'NONE',  ( 1.000000000000000000, 0.000000000000000000, 0.000000000000000000 ) ) ;
#7004=LINE ( 'NONE', #9372, #7542 ) ;
#7009=DIRECTION ( 'NONE',  ( -0.000000000000000000, 1.000000000000000000, 0.000000000000000000 ) ) ;
#7019=CARTESIAN_POINT ( 'NONE',  ( -63.50000000000002842, 17.53993994372674692, -17.50000000000002487 ) ) ;
#7033=CARTESIAN_POINT ( 'NONE',  ( -76.50000000000002842, 19.53993994372674337, 9.999999999999998224 ) ) ;
#7035=CARTESIAN_POINT ( 'NONE',  ( 14.00000000000004086, 64.51493994372674479, 15.00000000000104983 ) ) ;
#7039=EDGE_LOOP ( 'NONE', ( #10795, #10834 ) ) ;
#7042=ORIENTED_EDGE ( 'NONE', *, *, #8760, .T. ) ;
#7044=EDGE_LOOP ( 'NONE', ( #11648, #6838 ) ) ;
#7045=CARTESIAN_POINT ( 'NONE',  ( 14.00000000000004086, 59.53993994372674337, 13.30000000000105231 ) ) ;
#7050=CARTESIAN_POINT ( 'NONE',  ( 200.1062858801516597, 33.86394065090269123, 10.00000000000000533 ) ) ;
#7053=ORIENTED_EDGE ( 'NONE', *, *, #1398, .F. ) ;
#7063=ORIENTED_EDGE ( 'NONE', *, *, #7583, .F. ) ;
#7066=DIRECTION ( 'NONE',  ( -0.000000000000000000, -0.000000000000000000, 1.000000000000000000 ) ) ;
#7074=AXIS2_PLACEMENT_3D ( 'NONE', #6903, #10369, #8097 ) ;
#7075=DIRECTION ( 'NONE',  ( 0.000000000000000000, 0.000000000000000000, -1.000000000000000000 ) ) ;
#7076=CARTESIAN_POINT ( 'NONE',  ( -63.50000000000002842, 19.53993994372674692, -17.50000000000002487 ) ) ;
#7094=EDGE_CURVE ( 'NONE', #6265, #10437, #10234, .T. ) ;
#7102=CIRCLE ( 'NONE', #8610, 5.000000000000004441 ) ;
#7112=DIRECTION ( 'NONE',  ( 0.000000000000000000, 0.000000000000000000, -1.000000000000000000 ) ) ;
#7115=DIRECTION ( 'NONE',  ( -1.000000000000000000, 0.000000000000000000, -0.000000000000000000 ) ) ;
#7117=CIRCLE ( 'NONE', #5599, 1.699999999999993072 ) ;
#7120=ORIENTED_EDGE ( 'NONE', *, *, #13360, .F. ) ;
#7125=CARTESIAN_POINT ( 'NONE',  ( -85.99999999999994316, 62.13993994372673768, 15.00000000000174794 ) ) ;
#7127=ADVANCED_FACE ( 'NONE', ( #13533 ), #6692, .F. ) ;
#7131=EDGE_LOOP ( 'NONE', ( #337, #11198, #11234, #3434 ) ) ;
#7136=CARTESIAN_POINT ( 'NONE',  ( 64.00000000000005684, 59.53993994372674337, 15.00000000000070166 ) ) ;
#7139=EDGE_CURVE ( 'NONE', #470, #3955, #11866, .T. ) ;
#7143=ORIENTED_EDGE ( 'NONE', *, *, #1114, .F. ) ;
#7151=ORIENTED_EDGE ( 'NONE', *, *, #4463, .F. ) ;
#7156=VECTOR ( 'NONE', #14891, 1000.000000000000000 ) ;
#7159=ORIENTED_EDGE ( 'NONE', *, *, #5828, .T. ) ;
#7167=AXIS2_PLACEMENT_3D ( 'NONE', #759, #10412, #10561 ) ;
#7174=EDGE_LOOP ( 'NONE', ( #3580, #6115, #9982, #10506, #10000 ) ) ;
#7180=EDGE_CURVE ( 'NONE', #8016, #10578, #11616, .T. ) ;
#7185=AXIS2_PLACEMENT_3D ( 'NONE', #912, #10557, #1941 ) ;
#7186=CARTESIAN_POINT ( 'NONE',  ( -85.99999999999994316, 59.53993994372674337, 15.00000000000174794 ) ) ;
#7191=FACE_BOUND ( 'NONE', #2907, .T. ) ;
#7199=FILL_AREA_STYLE ('',( #2361 ) ) ;
#7202=DIRECTION ( 'NONE',  ( 0.000000000000000000, 0.000000000000000000, 1.000000000000000000 ) ) ;
#7204=EDGE_CURVE ( 'NONE', #9977, #11227, #11366, .T. ) ;
#7207=DIRECTION ( 'NONE',  ( 0.000000000000000000, -1.000000000000000000, 0.000000000000000000 ) ) ;
#7212=DIRECTION ( 'NONE',  ( 0.000000000000000000, 0.000000000000000000, -1.000000000000000000 ) ) ;
#7213=CARTESIAN_POINT ( 'NONE',  ( 64.00000000000005684, 64.51493994372674479, 15.00000000000070166 ) ) ;
#7216=DIRECTION ( 'NONE',  ( 0.000000000000000000, -0.000000000000000000, 1.000000000000000000 ) ) ;
#7217=EDGE_CURVE ( 'NONE', #2296, #4912, #8107, .T. ) ;
#7222=( NAMED_UNIT ( * ) PLANE_ANGLE_UNIT ( ) SI_UNIT ( $, .RADIAN. ) );
#7223=EDGE_CURVE ( 'NONE', #2412, #10382, #7346, .T. ) ;
#7224=ORIENTED_EDGE ( 'NONE', *, *, #13117, .T. ) ;
#7230=ORIENTED_EDGE ( 'NONE', *, *, #5370, .F. ) ;
#7238=ORIENTED_EDGE ( 'NONE', *, *, #13234, .F. ) ;
#7243=DIRECTION ( 'NONE',  ( -0.000000000000000000, -8.673617379884035472E-17, 1.000000000000000000 ) ) ;
#7244=EDGE_CURVE ( 'NONE', #5951, #10303, #13836, .T. ) ;
#7249=CARTESIAN_POINT ( 'NONE',  ( 194.0000000000000568, 59.53993994372674337, 20.00000000000000355 ) ) ;
#7251=ORIENTED_EDGE ( 'NONE', *, *, #10593, .F. ) ;
#7256=FACE_OUTER_BOUND ( 'NONE', #7950, .T. ) ;
#7259=CARTESIAN_POINT ( 'NONE',  ( 164.0000000000000568, 62.13993994372673768, 13.29999999999999538 ) ) ;
#7265=ORIENTED_EDGE ( 'NONE', *, *, #10773, .F. ) ;
#7273=DIRECTION ( 'NONE',  ( 0.000000000000000000, -1.000000000000000000, 0.000000000000000000 ) ) ;
#7275=VERTEX_POINT ( 'NONE', #10621 ) ;
#7281=ORIENTED_EDGE ( 'NONE', *, *, #14175, .F. ) ;
#7284=ORIENTED_EDGE ( 'NONE', *, *, #8741, .F. ) ;
#7286=DIRECTION ( 'NONE',  ( 0.000000000000000000, 0.000000000000000000, -1.000000000000000000 ) ) ;
#7289=CIRCLE ( 'NONE', #9296, 1.700000000000000178 ) ;
#7295=EDGE_LOOP ( 'NONE', ( #10877, #7305 ) ) ;
#7305=ORIENTED_EDGE ( 'NONE', *, *, #7204, .F. ) ;
#7308=CARTESIAN_POINT ( 'NONE',  ( -108.0000000000000568, 64.53993994372673626, 10.00000000000000178 ) ) ;
#7315=AXIS2_PLACEMENT_3D ( 'NONE', #4223, #7809, #2978 ) ;
#7330=CARTESIAN_POINT ( 'NONE',  ( 190.5000000000000568, 17.53993994372674692, -17.50000000000002487 ) ) ;
#7331=CARTESIAN_POINT ( 'NONE',  ( 64.00000000000005684, 64.53993994372673626, 15.00000000000070166 ) ) ;
#7333=LINE ( 'NONE', #1307, #4957 ) ;
#7335=DIRECTION ( 'NONE',  ( 0.000000000000000000, 1.000000000000000000, 0.000000000000000000 ) ) ;
#7346=CIRCLE ( 'NONE', #10565, 3.524999999999998579 ) ;
#7347=EDGE_LOOP ( 'NONE', ( #9765, #5857, #13236, #5992 ) ) ;
#7352=CARTESIAN_POINT ( 'NONE',  ( 115.7000000000000597, 62.13993994372673768, 15.00000000000035172 ) ) ;
#7360=FACE_OUTER_BOUND ( 'NONE', #8611, .T. ) ;
#7361=ORIENTED_EDGE ( 'NONE', *, *, #15375, .T. ) ;
#7363=ORIENTED_EDGE ( 'NONE', *, *, #889, .F. ) ;
#7366=AXIS2_PLACEMENT_3D ( 'NONE', #614, #10265, #6491 ) ;
#7368=LINE ( 'NONE', #1183, #10798 ) ;
#7369=CARTESIAN_POINT ( 'NONE',  ( 177.5000000000000853, 17.53993994372674692, -17.50000000000002487 ) ) ;
#7372=FACE_OUTER_BOUND ( 'NONE', #5056, .T. ) ;
#7376=CARTESIAN_POINT ( 'NONE',  ( 190.5000000000000568, 19.53993994372674692, -17.50000000000002487 ) ) ;
#7378=EDGE_LOOP ( 'NONE', ( #14938, #1616, #11470, #7682 ) ) ;
#7380=CARTESIAN_POINT ( 'NONE',  ( -85.99999999999994316, 62.13993994372673768, 15.00000000000174794 ) ) ;
#7391=AXIS2_PLACEMENT_3D ( 'NONE', #5198, #5352, #1473 ) ;
#7401=CARTESIAN_POINT ( 'NONE',  ( 64.00000000000005684, 56.53993994372675047, 16.70000000000069562 ) ) ;
#7413=AXIS2_PLACEMENT_3D ( 'NONE', #1405, #5360, #6238 ) ;
#7415=CARTESIAN_POINT ( 'NONE',  ( 185.1062858801516882, 55.86394065090267702, 18.00000000000000355 ) ) ;
#7416=EDGE_CURVE ( 'NONE', #163, #2412, #14389, .T. ) ;
#7417=EDGE_CURVE ( 'NONE', #2673, #2210, #9574, .T. ) ;
#7418=CARTESIAN_POINT ( 'NONE',  ( 114.0000000000000568, 64.53993994372673626, 15.00000000000035172 ) ) ;
#7421=ORIENTED_EDGE ( 'NONE', *, *, #10976, .T. ) ;
#7432=TOROIDAL_SURFACE ( 'NONE', #4903, 6.999999999999991118, 2.000000000000000000 ) ;
#7440=ORIENTED_EDGE ( 'NONE', *, *, #3383, .T. ) ;
#7444=AXIS2_PLACEMENT_3D ( 'NONE', #11502, #11574, #4299 ) ;
#7445=DIRECTION ( 'NONE',  ( 0.000000000000000000, 0.000000000000000000, -1.000000000000000000 ) ) ;
#7446=ORIENTED_EDGE ( 'NONE', *, *, #13549, .T. ) ;
#7451=CARTESIAN_POINT ( 'NONE',  ( 14.00000000000004086, 62.13993994372673768, 15.00000000000104983 ) ) ;
#7452=AXIS2_PLACEMENT_3D ( 'NONE', #8969, #12889, #1994 ) ;
#7458=ORIENTED_EDGE ( 'NONE', *, *, #7991, .F. ) ;
#7461=CARTESIAN_POINT ( 'NONE',  ( 14.00000000000004086, 64.53993994372673626, 15.00000000000104983 ) ) ;
#7464=ADVANCED_FACE ( 'NONE', ( #2401 ), #4856, .F. ) ;
#7465=FACE_BOUND ( 'NONE', #6355, .T. ) ;
#7475=CIRCLE ( 'NONE', #15011, 1.699999999999993072 ) ;
#7482=CARTESIAN_POINT ( 'NONE',  ( -85.99999999999994316, 62.13993994372673768, 18.50000000000175149 ) ) ;
#7498=DIRECTION ( 'NONE',  ( -0.000000000000000000, -0.000000000000000000, -1.000000000000000000 ) ) ;
#7505=DIRECTION ( 'NONE',  ( 1.000000000000000000, 0.000000000000000000, 0.000000000000000000 ) ) ;
#7516=DIRECTION ( 'NONE',  ( 8.659560562354932858E-17, 0.7071067811865474617, -0.7071067811865474617 ) ) ;
#7523=ORIENTED_EDGE ( 'NONE', *, *, #14249, .F. ) ;
#7524=DIRECTION ( 'NONE',  ( 0.000000000000000000, 1.156482317317871478E-16, -1.000000000000000000 ) ) ;
#7532=VERTEX_POINT ( 'NONE', #12564 ) ;
#7541=AXIS2_PLACEMENT_3D ( 'NONE', #8116, #12903, #14237 ) ;
#7542=VECTOR ( 'NONE', #11892, 1000.000000000000000 ) ;
#7547=FACE_BOUND ( 'NONE', #1340, .T. ) ;
#7556=CIRCLE ( 'NONE', #13069, 1.699999999999994849 ) ;
#7564=CARTESIAN_POINT ( 'NONE',  ( 194.0000000000000568, 59.53993994372674337, 10.00000000000000178 ) ) ;
#7567=CARTESIAN_POINT ( 'NONE',  ( -70.00000000000000000, 17.53993994372673981, -12.49999999999999467 ) ) ;
#7572=ORIENTED_EDGE ( 'NONE', *, *, #12429, .T. ) ;
#7573=AXIS2_PLACEMENT_3D ( 'NONE', #9292, #15192, #1068 ) ;
#7577=DIRECTION ( 'NONE',  ( 0.000000000000000000, -1.000000000000000000, 0.000000000000000000 ) ) ;
#7579=CARTESIAN_POINT ( 'NONE',  ( 224.0000000000000853, 19.53993994372674337, 24.99999999999999645 ) ) ;
#7583=EDGE_CURVE ( 'NONE', #61, #259, #6358, .T. ) ;
#7608=EDGE_CURVE ( 'NONE', #2275, #3552, #2716, .T. ) ;
#7612=CIRCLE ( 'NONE', #13894, 3.500000000000001332 ) ;
#7624=VECTOR ( 'NONE', #15601, 1000.000000000000114 ) ;
#7638=CARTESIAN_POINT ( 'NONE',  ( -35.99999999999995026, 62.13993994372673768, 15.00000000000139977 ) ) ;
#7642=EDGE_CURVE ( 'NONE', #2814, #15158, #15608, .T. ) ;
#7644=AXIS2_PLACEMENT_3D ( 'NONE', #6018, #14525, #11867 ) ;
#7651=DIRECTION ( 'NONE',  ( 0.000000000000000000, 0.000000000000000000, 1.000000000000000000 ) ) ;
#7652=ORIENTED_EDGE ( 'NONE', *, *, #2238, .T. ) ;
#7654=DIRECTION ( 'NONE',  ( 3.965082230804130220E-16, 0.000000000000000000, 1.000000000000000000 ) ) ;
#7656=CARTESIAN_POINT ( 'NONE',  ( 164.0000000000000568, 56.53993994372675047, 15.00000000000000355 ) ) ;
#7664=CARTESIAN_POINT ( 'NONE',  ( 195.1062858801516597, 40.86394065090267702, -219.0000000000000853 ) ) ;
#7665=DIRECTION ( 'NONE',  ( 3.965082230804130220E-16, 0.000000000000000000, -1.000000000000000000 ) ) ;
#7669=ORIENTED_EDGE ( 'NONE', *, *, #4922, .F. ) ;
#7673=ORIENTED_EDGE ( 'NONE', *, *, #6277, .F. ) ;
#7682=ORIENTED_EDGE ( 'NONE', *, *, #6218, .F. ) ;
#7689=FACE_OUTER_BOUND ( 'NONE', #8125, .T. ) ;
#7697=LINE ( 'NONE', #12560, #10857 ) ;
#7698=FACE_OUTER_BOUND ( 'NONE', #10538, .T. ) ;
#7702=ADVANCED_FACE ( 'NONE', ( #9269 ), #3180, .F. ) ;
#7705=ADVANCED_FACE ( 'NONE', ( #8176 ), #13993, .F. ) ;
#7707=FACE_OUTER_BOUND ( 'NONE', #309, .T. ) ;
#7713=ORIENTED_EDGE ( 'NONE', *, *, #2507, .T. ) ;
#7734=ORIENTED_EDGE ( 'NONE', *, *, #4024, .F. ) ;
#7737=CARTESIAN_POINT ( 'NONE',  ( 224.0000000000000853, 59.53993994372674337, 25.00000000000000000 ) ) ;
#7739=DIRECTION ( 'NONE',  ( -0.000000000000000000, 1.000000000000000000, -0.000000000000000000 ) ) ;
#7742=CIRCLE ( 'NONE', #11766, 3.499999999999999556 ) ;
#7745=LINE ( 'NONE', #7664, #15203 ) ;
#7750=ADVANCED_FACE ( 'NONE', ( #15163 ), #11548, .F. ) ;
#7755=ORIENTED_EDGE ( 'NONE', *, *, #9956, .F. ) ;
#7760=ORIENTED_EDGE ( 'NONE', *, *, #2163, .T. ) ;
#7765=FACE_OUTER_BOUND ( 'NONE', #2404, .T. ) ;
#7770=ORIENTED_EDGE ( 'NONE', *, *, #10282, .T. ) ;
#7774=FACE_OUTER_BOUND ( 'NONE', #14609, .T. ) ;
#7778=VECTOR ( 'NONE', #3775, 1000.000000000000114 ) ;
#7779=DIRECTION ( 'NONE',  ( 1.000000000000000000, 0.000000000000000000, 0.000000000000000000 ) ) ;
#7785=ADVANCED_FACE ( 'NONE', ( #15314 ), #2145, .F. ) ;
#7797=CARTESIAN_POINT ( 'NONE',  ( -85.99999999999994316, 64.53993994372673626, 15.00000000000174794 ) ) ;
#7806=AXIS2_PLACEMENT_3D ( 'NONE', #3999, #10094, #7654 ) ;
#7809=DIRECTION ( 'NONE',  ( -0.000000000000000000, 1.000000000000000000, 1.156482317317871725E-16 ) ) ;
#7812=AXIS2_PLACEMENT_3D ( 'NONE', #9105, #13906, #5303 ) ;
#7815=FACE_OUTER_BOUND ( 'NONE', #11963, .T. ) ;
#7820=AXIS2_PLACEMENT_3D ( 'NONE', #8113, #12898, #891 ) ;
#7822=AXIS2_PLACEMENT_3D ( 'NONE', #11777, #3170, #9408 ) ;
#7828=CARTESIAN_POINT ( 'NONE',  ( 184.0000000000000568, 17.53993994372673271, 47.49999999999997868 ) ) ;
#7843=ORIENTED_EDGE ( 'NONE', *, *, #6986, .F. ) ;
#7848=ORIENTED_EDGE ( 'NONE', *, *, #3820, .F. ) ;
#7851=AXIS2_PLACEMENT_3D ( 'NONE', #10038, #5375, #3006 ) ;
#7856=AXIS2_PLACEMENT_3D ( 'NONE', #2830, #12368, #7651 ) ;
#7857=ORIENTED_EDGE ( 'NONE', *, *, #9621, .F. ) ;
#7859=EDGE_CURVE ( 'NONE', #5720, #10088, #3644, .T. ) ;
#7860=CARTESIAN_POINT ( 'NONE',  ( 14.00000000000004086, 64.53993994372673626, 15.00000000000104983 ) ) ;
#7863=EDGE_CURVE ( 'NONE', #10197, #701, #13164, .T. ) ;
#7864=DIRECTION ( 'NONE',  ( 0.000000000000000000, 0.000000000000000000, -1.000000000000000000 ) ) ;
#7866=VECTOR ( 'NONE', #8917, 1000.000000000000000 ) ;
#7869=CARTESIAN_POINT ( 'NONE',  ( -110.0000000000000426, 56.53993994372675047, 13.00000000000000178 ) ) ;
#7871=DIRECTION ( 'NONE',  ( 0.000000000000000000, -1.000000000000000000, -1.156482317317871725E-16 ) ) ;
#7876=VECTOR ( 'NONE', #10675, 1000.000000000000000 ) ;
#7882=CARTESIAN_POINT ( 'NONE',  ( -108.0000000000000568, 26.39124795404934076, 0.000000000000000000 ) ) ;
#7887=CARTESIAN_POINT ( 'NONE',  ( -63.50000000000002842, 17.53993994372674692, -17.50000000000002487 ) ) ;
#7890=EDGE_LOOP ( 'NONE', ( #7941, #8523, #11641, #527 ) ) ;
#7891=CARTESIAN_POINT ( 'NONE',  ( -110.0000000000000426, 22.53993994372673981, 13.00000000000000178 ) ) ;
#7895=CARTESIAN_POINT ( 'NONE',  ( -70.00000000000000000, 17.53993994372673271, 48.99999999999997158 ) ) ;
#7901=ADVANCED_FACE ( 'NONE', ( #13340 ), #147, .T. ) ;
#7905=CARTESIAN_POINT ( 'NONE',  ( 14.00000000000004086, 59.53993994372674337, 15.00000000000104983 ) ) ;
#7913=ORIENTED_EDGE ( 'NONE', *, *, #8029, .T. ) ;
#7920=ORIENTED_EDGE ( 'NONE', *, *, #8481, .F. ) ;
#7923=DIRECTION ( 'NONE',  ( 0.000000000000000000, 0.000000000000000000, 1.000000000000000000 ) ) ;
#7932=ORIENTED_EDGE ( 'NONE', *, *, #1908, .T. ) ;
#7935=AXIS2_PLACEMENT_3D ( 'NONE', #12614, #9002, #13718 ) ;
#7937=PLANE ( 'NONE',  #5456 ) ;
#7939=CIRCLE ( 'NONE', #1104, 1.700000000000007061 ) ;
#7940=DIRECTION ( 'NONE',  ( 0.000000000000000000, -0.000000000000000000, -1.000000000000000000 ) ) ;
#7941=ORIENTED_EDGE ( 'NONE', *, *, #7416, .F. ) ;
#7947=ADVANCED_FACE ( 'NONE', ( #7372 ), #12165, .F. ) ;
#7950=EDGE_LOOP ( 'NONE', ( #3844, #11036, #11992, #11774 ) ) ;
#7956=PLANE ( 'NONE',  #9141 ) ;
#7979=CARTESIAN_POINT ( 'NONE',  ( 200.1062858801516597, 40.86394065090267702, 16.00000000000001421 ) ) ;
#7980=FACE_OUTER_BOUND ( 'NONE', #3654, .T. ) ;
#7985=EDGE_CURVE ( 'NONE', #6589, #5209, #13109, .T. ) ;
#7989=CARTESIAN_POINT ( 'NONE',  ( 200.1062858801516597, 33.86394065090269123, 12.00000000000001066 ) ) ;
#7990=DIRECTION ( 'NONE',  ( 0.000000000000000000, -1.000000000000000000, 0.000000000000000000 ) ) ;
#7991=EDGE_CURVE ( 'NONE', #9297, #10399, #2601, .T. ) ;
#7995=SHAPE_DEFINITION_REPRESENTATION ( #3232, #3806 ) ;
#7999=AXIS2_PLACEMENT_3D ( 'NONE', #11843, #6160, #7115 ) ;
#8000=DIRECTION ( 'NONE',  ( 1.000000000000000000, 0.000000000000000000, 0.000000000000000000 ) ) ;
#8002=EDGE_CURVE ( 'NONE', #6470, #12466, #9892, .T. ) ;
#8005=ORIENTED_EDGE ( 'NONE', *, *, #12091, .T. ) ;
#8008=ORIENTED_EDGE ( 'NONE', *, *, #4797, .F. ) ;
#8009=LINE ( 'NONE', #6511, #14112 ) ;
#8010=DIRECTION ( 'NONE',  ( -0.000000000000000000, 1.000000000000000000, -0.000000000000000000 ) ) ;
#8012=LINE ( 'NONE', #4434, #11258 ) ;
#8016=VERTEX_POINT ( 'NONE', #12240 ) ;
#8029=EDGE_CURVE ( 'NONE', #5720, #10245, #2620, .T. ) ;
#8031=AXIS2_PLACEMENT_3D ( 'NONE', #2901, #6537, #8803 ) ;
#8033=CARTESIAN_POINT ( 'NONE',  ( 164.0000000000000568, 64.53993994372673626, 11.47500000000000320 ) ) ;
#8034=EDGE_CURVE ( 'NONE', #5037, #15478, #14830, .T. ) ;
#8044=ORIENTED_EDGE ( 'NONE', *, *, #14903, .F. ) ;
#8057=EDGE_CURVE ( 'NONE', #12734, #10742, #8644, .T. ) ;
#8065=CARTESIAN_POINT ( 'NONE',  ( 14.00000000000004086, 56.53993994372675047, 16.70000000000105089 ) ) ;
#8066=DIRECTION ( 'NONE',  ( 0.000000000000000000, 0.000000000000000000, -1.000000000000000000 ) ) ;
#8079=VECTOR ( 'NONE', #3702, 1000.000000000000000 ) ;
#8084=AXIS2_PLACEMENT_3D ( 'NONE', #1911, #954, #12883 ) ;
#8088=ORIENTED_EDGE ( 'NONE', *, *, #13659, .T. ) ;
#8089=CARTESIAN_POINT ( 'NONE',  ( 200.1062858801516597, 35.86394065090269123, 12.00000000000001066 ) ) ;
#8090=DIRECTION ( 'NONE',  ( 0.000000000000000000, -1.000000000000000000, -1.486905836551548832E-16 ) ) ;
#8097=DIRECTION ( 'NONE',  ( 1.000000000000000000, 0.000000000000000000, 0.000000000000000000 ) ) ;
#8101=FACE_OUTER_BOUND ( 'NONE', #11339, .T. ) ;
#8105=CIRCLE ( 'NONE', #1019, 1.499999999999994449 ) ;
#8107=CIRCLE ( 'NONE', #1266, 1.700000000000007061 ) ;
#8112=EDGE_LOOP ( 'NONE', ( #3808, #9971, #8088, #2951 ) ) ;
#8113=CARTESIAN_POINT ( 'NONE',  ( -63.50000000000002842, 17.53993994372673271, 52.49999999999997868 ) ) ;
#8115=VECTOR ( 'NONE', #2044, 1000.000000000000000 ) ;
#8116=CARTESIAN_POINT ( 'NONE',  ( -85.99999999999994316, 64.51493994372674479, 15.00000000000174794 ) ) ;
#8119=LINE ( 'NONE', #8033, #14908 ) ;
#8125=EDGE_LOOP ( 'NONE', ( #5431, #11725, #15039, #4180, #12004, #8707, #14094, #5893 ) ) ;
#8127=FACE_OUTER_BOUND ( 'NONE', #3799, .T. ) ;
#8128=ORIENTED_EDGE ( 'NONE', *, *, #2591, .T. ) ;
#8130=VERTEX_POINT ( 'NONE', #10196 ) ;
#8135=FACE_OUTER_BOUND ( 'NONE', #5926, .T. ) ;
#8144=DIRECTION ( 'NONE',  ( 0.000000000000000000, 0.000000000000000000, 1.000000000000000000 ) ) ;
#8145=CARTESIAN_POINT ( 'NONE',  ( -85.99999999999994316, 59.53993994372674337, 15.00000000000174794 ) ) ;
#8147=DIRECTION ( 'NONE',  ( 0.000000000000000000, 0.000000000000000000, 1.000000000000000000 ) ) ;
#8153=ORIENTED_EDGE ( 'NONE', *, *, #1829, .F. ) ;
#8155=CARTESIAN_POINT ( 'NONE',  ( 164.0000000000000568, 59.53993994372674337, 13.29999999999999538 ) ) ;
#8164=VECTOR ( 'NONE', #220, 1000.000000000000000 ) ;
#8176=FACE_OUTER_BOUND ( 'NONE', #4857, .T. ) ;
#8177=CIRCLE ( 'NONE', #13947, 1.700000000000007061 ) ;
#8178=FACE_OUTER_BOUND ( 'NONE', #8582, .T. ) ;
#8179=EDGE_LOOP ( 'NONE', ( #2636, #6766, #6937, #6669 ) ) ;
#8180=ADVANCED_FACE ( 'NONE', ( #4253, #12702 ), #11531, .F. ) ;
#8183=DIRECTION ( 'NONE',  ( -0.000000000000000000, 1.000000000000000000, 1.156482317317871725E-16 ) ) ;
#8184=EDGE_LOOP ( 'NONE', ( #12436, #1805, #14450, #4367 ) ) ;
#8188=AXIS2_PLACEMENT_3D ( 'NONE', #14972, #10334, #6559 ) ;
#8189=ORIENTED_EDGE ( 'NONE', *, *, #4874, .T. ) ;
#8202=CARTESIAN_POINT ( 'NONE',  ( -35.99999999999995026, 64.53993994372673626, 15.00000000000139977 ) ) ;
#8215=CARTESIAN_POINT ( 'NONE',  ( 114.0000000000000568, 64.53993994372673626, 18.52500000000035385 ) ) ;
#8222=CIRCLE ( 'NONE', #9729, 1.699999999999993072 ) ;
#8227=ORIENTED_EDGE ( 'NONE', *, *, #15166, .T. ) ;
#8235=ORIENTED_EDGE ( 'NONE', *, *, #13462, .F. ) ;
#8240=DIRECTION ( 'NONE',  ( 0.000000000000000000, 0.7071067811864985009, 0.7071067811865965336 ) ) ;
#8242=EDGE_LOOP ( 'NONE', ( #7361, #8598, #487, #8153 ) ) ;
#8243=ORIENTED_EDGE ( 'NONE', *, *, #10623, .T. ) ;
#8250=VERTEX_POINT ( 'NONE', #15063 ) ;
#8252=DIRECTION ( 'NONE',  ( 0.000000000000000000, -1.486905836551548832E-16, 1.000000000000000000 ) ) ;
#8261=EDGE_LOOP ( 'NONE', ( #15148, #5447, #1424, #6563 ) ) ;
#8274=ADVANCED_FACE ( 'NONE', ( #353 ), #2833, .F. ) ;
#8276=EDGE_CURVE ( 'NONE', #701, #10197, #11182, .T. ) ;
#8279=EDGE_LOOP ( 'NONE', ( #6215, #5410, #14643, #1635 ) ) ;
#8289=ADVANCED_FACE ( 'NONE', ( #7815 ), #8660, .F. ) ;
#8297=ORIENTED_EDGE ( 'NONE', *, *, #4994, .F. ) ;
#8299=VERTEX_POINT ( 'NONE', #8994 ) ;
#8301=CARTESIAN_POINT ( 'NONE',  ( 64.00000000000005684, 64.51493994372674479, 11.50000000000069811 ) ) ;
#8307=PRODUCT_DEFINITION_FORMATION_WITH_SPECIFIED_SOURCE ( 'ANY', '', #9174, .NOT_KNOWN. ) ;
#8318=CYLINDRICAL_SURFACE ( 'NONE', #10319, 1.499999999999997780 ) ;
#8321=EDGE_LOOP ( 'NONE', ( #3399, #15108, #3334, #1045 ) ) ;
#8323=ADVANCED_FACE ( 'NONE', ( #10247 ), #8832, .F. ) ;
#8325=AXIS2_PLACEMENT_3D ( 'NONE', #968, #6994, #6840 ) ;
#8327=SURFACE_STYLE_FILL_AREA ( #15317 ) ;
#8330=CARTESIAN_POINT ( 'NONE',  ( 114.0000000000000568, 64.53993994372673626, 13.30000000000035776 ) ) ;
#8332=DIRECTION ( 'NONE',  ( 0.000000000000000000, 0.000000000000000000, -1.000000000000000000 ) ) ;
#8339=AXIS2_PLACEMENT_3D ( 'NONE', #5046, #14581, #9786 ) ;
#8340=AXIS2_PLACEMENT_3D ( 'NONE', #716, #11786, #641 ) ;
#8344=VECTOR ( 'NONE', #15312, 1000.000000000000000 ) ;
#8356=FACE_BOUND ( 'NONE', #3816, .T. ) ;
#8357=ORIENTED_EDGE ( 'NONE', *, *, #1026, .T. ) ;
#8358=ORIENTED_EDGE ( 'NONE', *, *, #11075, .F. ) ;
#8361=CARTESIAN_POINT ( 'NONE',  ( 190.5000000000000568, 19.53993994372674337, 9.999999999999998224 ) ) ;
#8372=CARTESIAN_POINT ( 'NONE',  ( 184.0000000000000568, 17.53993994372673981, -10.99999999999999822 ) ) ;
#8376=ORIENTED_EDGE ( 'NONE', *, *, #4567, .T. ) ;
#8382=DIRECTION ( 'NONE',  ( -0.000000000000000000, -0.000000000000000000, -1.000000000000000000 ) ) ;
#8389=CIRCLE ( 'NONE', #12902, 1.699999999999993072 ) ;
#8395=VERTEX_POINT ( 'NONE', #5666 ) ;
#8401=AXIS2_PLACEMENT_3D ( 'NONE', #6225, #2669, #14655 ) ;
#8408=CIRCLE ( 'NONE', #2340, 1.499999999999994449 ) ;
#8427=EDGE_CURVE ( 'NONE', #7532, #9928, #3990, .T. ) ;
#8431=DIRECTION ( 'NONE',  ( 0.000000000000000000, 1.000000000000000000, 0.000000000000000000 ) ) ;
#8434=CARTESIAN_POINT ( 'NONE',  ( 190.5000000000000853, 19.53993994372673626, 52.49999999999997868 ) ) ;
#8439=ORIENTED_EDGE ( 'NONE', *, *, #889, .T. ) ;
#8441=DIRECTION ( 'NONE',  ( -0.000000000000000000, 1.000000000000000000, -0.000000000000000000 ) ) ;
#8447=CARTESIAN_POINT ( 'NONE',  ( -110.0000000000000426, 59.53993994372674337, 25.00000000000000000 ) ) ;
#8451=DIRECTION ( 'NONE',  ( -0.000000000000000000, 1.000000000000000000, 1.156482317317871725E-16 ) ) ;
#8459=DIRECTION ( 'NONE',  ( -0.000000000000000000, 1.000000000000000000, 1.156482317317871725E-16 ) ) ;
#8462=EDGE_CURVE ( 'NONE', #1700, #1434, #842, .T. ) ;
#8463=ORIENTED_EDGE ( 'NONE', *, *, #253, .F. ) ;
#8470=ORIENTED_EDGE ( 'NONE', *, *, #1796, .F. ) ;
#8471=EDGE_CURVE ( 'NONE', #4243, #11151, #10553, .T. ) ;
#8475=ORIENTED_EDGE ( 'NONE', *, *, #2911, .T. ) ;
#8478=CARTESIAN_POINT ( 'NONE',  ( -110.0000000000000426, 22.53993994372673981, 13.00000000000000178 ) ) ;
#8480=ORIENTED_EDGE ( 'NONE', *, *, #13174, .F. ) ;
#8481=EDGE_CURVE ( 'NONE', #6899, #411, #11709, .T. ) ;
#8482=FACE_OUTER_BOUND ( 'NONE', #11125, .T. ) ;
#8489=EDGE_LOOP ( 'NONE', ( #5974, #2389, #6035, #3908 ) ) ;
#8495=DIRECTION ( 'NONE',  ( 0.000000000000000000, 1.000000000000000000, 0.000000000000000000 ) ) ;
#8502=CARTESIAN_POINT ( 'NONE',  ( -110.0000000000000426, 19.53993994372674337, 9.999999999999998224 ) ) ;
#8509=ORIENTED_EDGE ( 'NONE', *, *, #3722, .T. ) ;
#8512=DIRECTION ( 'NONE',  ( -0.000000000000000000, 1.000000000000000000, -0.000000000000000000 ) ) ;
#8514=CARTESIAN_POINT ( 'NONE',  ( 164.0000000000000568, 64.51493994372674479, 15.00000000000000355 ) ) ;
#8519=CARTESIAN_POINT ( 'NONE',  ( -63.50000000000002842, 17.53993994372673271, 52.49999999999997868 ) ) ;
#8522=LINE ( 'NONE', #119, #14872 ) ;
#8523=ORIENTED_EDGE ( 'NONE', *, *, #9809, .F. ) ;
#8524=DIRECTION ( 'NONE',  ( -1.000000000000000000, 0.000000000000000000, 0.000000000000000000 ) ) ;
#8528=PLANE ( 'NONE',  #4968 ) ;
#8529=DIRECTION ( 'NONE',  ( 0.000000000000000000, 0.000000000000000000, 1.000000000000000000 ) ) ;
#8531=EDGE_CURVE ( 'NONE', #1467, #299, #6860, .T. ) ;
#8543=VERTEX_POINT ( 'NONE', #3136 ) ;
#8551=EDGE_LOOP ( 'NONE', ( #7458, #370 ) ) ;
#8558=ORIENTED_EDGE ( 'NONE', *, *, #7583, .T. ) ;
#8562=VERTEX_POINT ( 'NONE', #5593 ) ;
#8572=CARTESIAN_POINT ( 'NONE',  ( -85.99999999999994316, 62.13993994372673768, 15.00000000000174794 ) ) ;
#8573=CIRCLE ( 'NONE', #7573, 1.700000000000001954 ) ;
#8582=EDGE_LOOP ( 'NONE', ( #6112, #490, #12473, #666 ) ) ;
#8589=CARTESIAN_POINT ( 'NONE',  ( -85.99999999999994316, 56.53993994372675047, 16.70000000000174012 ) ) ;
#8596=CIRCLE ( 'NONE', #10358, 3.500000000000004885 ) ;
#8598=ORIENTED_EDGE ( 'NONE', *, *, #5870, .T. ) ;
#8602=CARTESIAN_POINT ( 'NONE',  ( -110.0000000000000426, 19.53993994372674337, 9.999999999999998224 ) ) ;
#8610=AXIS2_PLACEMENT_3D ( 'NONE', #871, #10135, #2949 ) ;
#8611=EDGE_LOOP ( 'NONE', ( #926, #7760, #13456, #702 ) ) ;
#8623=DIRECTION ( 'NONE',  ( 0.000000000000000000, -1.000000000000000000, 0.000000000000000000 ) ) ;
#8626=VERTEX_POINT ( 'NONE', #6435 ) ;
#8632=VERTEX_POINT ( 'NONE', #10796 ) ;
#8644=CIRCLE ( 'NONE', #9910, 1.699999999999998401 ) ;
#8649=LINE ( 'NONE', #9912, #12156 ) ;
#8655=PLANE ( 'NONE',  #960 ) ;
#8660=CONICAL_SURFACE ( 'NONE', #10668, 3.525000000000000355, 0.7853981633974482790 ) ;
#8669=CARTESIAN_POINT ( 'NONE',  ( -35.99999999999995026, 64.53993994372673626, 15.00000000000139977 ) ) ;
#8679=EDGE_LOOP ( 'NONE', ( #2418, #1219 ) ) ;
#8680=LINE ( 'NONE', #6309, #4997 ) ;
#8683=CARTESIAN_POINT ( 'NONE',  ( 190.5000000000000568, 19.53993994372674337, 24.99999999999999645 ) ) ;
#8685=CARTESIAN_POINT ( 'NONE',  ( -35.99999999999995026, 64.53993994372673626, 15.00000000000139977 ) ) ;
#8689=ORIENTED_EDGE ( 'NONE', *, *, #1281, .T. ) ;
#8690=EDGE_CURVE ( 'NONE', #3509, #9250, #2260, .T. ) ;
#8701=LINE ( 'NONE', #5519, #4136 ) ;
#8702=CARTESIAN_POINT ( 'NONE',  ( -35.99999999999995026, 56.53993994372675047, 13.30000000000139870 ) ) ;
#8705=EDGE_LOOP ( 'NONE', ( #1751, #9941, #4537, #10470 ) ) ;
#8707=ORIENTED_EDGE ( 'NONE', *, *, #13225, .F. ) ;
#8708=DIRECTION ( 'NONE',  ( -0.000000000000000000, 1.000000000000000000, -0.000000000000000000 ) ) ;
#8711=DIRECTION ( 'NONE',  ( 0.000000000000000000, 0.000000000000000000, 1.000000000000000000 ) ) ;
#8712=AXIS2_PLACEMENT_3D ( 'NONE', #10299, #6830, #11642 ) ;
#8731=VERTEX_POINT ( 'NONE', #13913 ) ;
#8736=EDGE_CURVE ( 'NONE', #10088, #5037, #8009, .T. ) ;
#8738=CARTESIAN_POINT ( 'NONE',  ( 184.0000000000000568, 19.53993994372674337, -12.49999999999999467 ) ) ;
#8741=EDGE_CURVE ( 'NONE', #13912, #9198, #5803, .T. ) ;
#8760=EDGE_CURVE ( 'NONE', #4694, #8543, #7697, .T. ) ;
#8762=ORIENTED_EDGE ( 'NONE', *, *, #7985, .F. ) ;
#8767=EDGE_LOOP ( 'NONE', ( #4191, #5547 ) ) ;
#8769=CARTESIAN_POINT ( 'NONE',  ( -85.99999999999994316, 64.53993994372673626, 11.47500000000174758 ) ) ;
#8780=CARTESIAN_POINT ( 'NONE',  ( 64.00000000000005684, 64.53993994372673626, 13.30000000000070948 ) ) ;
#8786=EDGE_CURVE ( 'NONE', #12099, #470, #13356, .T. ) ;
#8793=EDGE_CURVE ( 'NONE', #10245, #2490, #14032, .T. ) ;
#8800=ORIENTED_EDGE ( 'NONE', *, *, #12696, .T. ) ;
#8803=DIRECTION ( 'NONE',  ( 0.000000000000000000, 0.000000000000000000, 1.000000000000000000 ) ) ;
#8804=ORIENTED_EDGE ( 'NONE', *, *, #2804, .F. ) ;
#8817=DIRECTION ( 'NONE',  ( 0.000000000000000000, 1.000000000000000000, 0.000000000000000000 ) ) ;
#8822=CARTESIAN_POINT ( 'NONE',  ( -70.00000000000000000, 19.53993994372673626, 47.49999999999997868 ) ) ;
#8824=FACE_OUTER_BOUND ( 'NONE', #1710, .T. ) ;
#8826=ORIENTED_EDGE ( 'NONE', *, *, #14111, .F. ) ;
#8828=ADVANCED_FACE ( 'NONE', ( #7980 ), #13600, .F. ) ;
#8829=ORIENTED_EDGE ( 'NONE', *, *, #2529, .T. ) ;
#8831=CONICAL_SURFACE ( 'NONE', #1755, 3.525000000000000355, 0.7853981633974482790 ) ;
#8832=PLANE ( 'NONE',  #7806 ) ;
#8833=LINE ( 'NONE', #8602, #9037 ) ;
#8837=CARTESIAN_POINT ( 'NONE',  ( 14.00000000000004086, 64.53993994372673626, 16.70000000000104734 ) ) ;
#8838=LINE ( 'NONE', #9947, #13514 ) ;
#8853=ORIENTED_EDGE ( 'NONE', *, *, #3852, .T. ) ;
#8856=ORIENTED_EDGE ( 'NONE', *, *, #12091, .F. ) ;
#8860=EDGE_CURVE ( 'NONE', #701, #9198, #1083, .T. ) ;
#8866=LINE ( 'NONE', #6500, #4393 ) ;
#8870=AXIS2_PLACEMENT_3D ( 'NONE', #10190, #4171, #9010 ) ;
#8882=DIRECTION ( 'NONE',  ( -0.000000000000000000, -1.000000000000000000, -0.000000000000000000 ) ) ;
#8887=ADVANCED_FACE ( 'NONE', ( #46 ), #15439, .F. ) ;
#8896=AXIS2_PLACEMENT_3D ( 'NONE', #10626, #9368, #2094 ) ;
#8898=EDGE_LOOP ( 'NONE', ( #9441, #14356, #7652, #12872 ) ) ;
#8907=LINE ( 'NONE', #13698, #5919 ) ;
#8913=ORIENTED_EDGE ( 'NONE', *, *, #7217, .F. ) ;
#8917=DIRECTION ( 'NONE',  ( -0.000000000000000000, -0.000000000000000000, 1.000000000000000000 ) ) ;
#8919=DIRECTION ( 'NONE',  ( -0.000000000000000000, -1.000000000000000000, -0.000000000000000000 ) ) ;
#8929=VERTEX_POINT ( 'NONE', #12021 ) ;
#8932=ORIENTED_EDGE ( 'NONE', *, *, #8276, .T. ) ;
#8937=PLANE ( 'NONE',  #12959 ) ;
#8966=DIRECTION ( 'NONE',  ( -0.000000000000000000, 1.000000000000000000, 0.000000000000000000 ) ) ;
#8969=CARTESIAN_POINT ( 'NONE',  ( 114.0000000000000568, 64.53993994372673626, 15.00000000000035172 ) ) ;
#8981=CARTESIAN_POINT ( 'NONE',  ( 200.1062858801516597, 40.86394065090267702, 12.00000000000001066 ) ) ;
#8982=FACE_BOUND ( 'NONE', #6013, .T. ) ;
#8989=AXIS2_PLACEMENT_3D ( 'NONE', #1521, #14774, #13513 ) ;
#8994=CARTESIAN_POINT ( 'NONE',  ( -110.0000000000000426, 19.53993994372674337, 24.99999999999999645 ) ) ;
#8995=LINE ( 'NONE', #432, #1339 ) ;
#8999=AXIS2_PLACEMENT_3D ( 'NONE', #6747, #560, #11480 ) ;
#9002=DIRECTION ( 'NONE',  ( -0.000000000000000000, 1.000000000000000000, -0.000000000000000000 ) ) ;
#9005=ORIENTED_EDGE ( 'NONE', *, *, #4922, .T. ) ;
#9010=DIRECTION ( 'NONE',  ( 0.000000000000000000, -0.000000000000000000, -1.000000000000000000 ) ) ;
#9014=CARTESIAN_POINT ( 'NONE',  ( 0.000000000000000000, 19.53993994372674337, 2.905405074819403421E-15 ) ) ;
#9026=ORIENTED_EDGE ( 'NONE', *, *, #5574, .T. ) ;
#9028=LINE ( 'NONE', #6742, #11885 ) ;
#9029=EDGE_CURVE ( 'NONE', #10578, #8562, #3346, .T. ) ;
#9037=VECTOR ( 'NONE', #4083, 1000.000000000000000 ) ;
#9040=DIRECTION ( 'NONE',  ( 0.000000000000000000, -1.000000000000000000, 0.000000000000000000 ) ) ;
#9056=PLANE ( 'NONE',  #11661 ) ;
#9063=ORIENTED_EDGE ( 'NONE', *, *, #10011, .T. ) ;
#9068=ORIENTED_EDGE ( 'NONE', *, *, #5870, .F. ) ;
#9080=EDGE_CURVE ( 'NONE', #14978, #13487, #10612, .T. ) ;
#9083=DIRECTION ( 'NONE',  ( 0.000000000000000000, 0.000000000000000000, -1.000000000000000000 ) ) ;
#9084=EDGE_LOOP ( 'NONE', ( #10792, #13275, #10047, #10111 ) ) ;
#9089=DIRECTION ( 'NONE',  ( -0.000000000000000000, 1.000000000000000000, 0.000000000000000000 ) ) ;
#9105=CARTESIAN_POINT ( 'NONE',  ( 114.0000000000000568, 64.53993994372673626, 15.00000000000035172 ) ) ;
#9106=ORIENTED_EDGE ( 'NONE', *, *, #5572, .F. ) ;
#9109=EDGE_CURVE ( 'NONE', #1434, #1700, #9614, .T. ) ;
#9110=CARTESIAN_POINT ( 'NONE',  ( 0.000000000000000000, 17.53993994372673981, 2.674108611355829274E-15 ) ) ;
#9119=EDGE_CURVE ( 'NONE', #5590, #6168, #10670, .T. ) ;
#9130=ORIENTED_EDGE ( 'NONE', *, *, #7416, .T. ) ;
#9132=FACE_OUTER_BOUND ( 'NONE', #3055, .T. ) ;
#9134=EDGE_CURVE ( 'NONE', #2673, #3949, #8522, .T. ) ;
#9140=ORIENTED_EDGE ( 'NONE', *, *, #7180, .F. ) ;
#9141=AXIS2_PLACEMENT_3D ( 'NONE', #7882, #12906, #6617 ) ;
#9145=ADVANCED_FACE ( 'NONE', ( #4658 ), #9487, .F. ) ;
#9146=VECTOR ( 'NONE', #1318, 1000.000000000000000 ) ;
#9163=DIRECTION ( 'NONE',  ( -0.000000000000000000, -1.000000000000000000, -0.000000000000000000 ) ) ;
#9164=CARTESIAN_POINT ( 'NONE',  ( 224.0000000000000853, 59.53993994372674337, 10.00000000000000178 ) ) ;
#9166=EDGE_LOOP ( 'NONE', ( #3993, #7363 ) ) ;
#9171=DIRECTION ( 'NONE',  ( 1.000000000000000000, 0.000000000000000000, 0.000000000000000000 ) ) ;
#9173=CARTESIAN_POINT ( 'NONE',  ( -34.29999999999994742, 62.13993994372673768, 15.00000000000139977 ) ) ;
#9174=PRODUCT ( 'Lower Fixed Bed Shear Blade', 'Lower Fixed Bed Shear Blade', '', ( #12548 ) ) ;
#9196=CIRCLE ( 'NONE', #14464, 2.000000000000001776 ) ;
#9198=VERTEX_POINT ( 'NONE', #11122 ) ;
#9199=CARTESIAN_POINT ( 'NONE',  ( -85.99999999999994316, 56.53993994372675047, 15.00000000000174794 ) ) ;
#9209=EDGE_CURVE ( 'NONE', #10379, #15150, #8105, .T. ) ;
#9210=ORIENTED_EDGE ( 'NONE', *, *, #4674, .T. ) ;
#9213=ORIENTED_EDGE ( 'NONE', *, *, #8471, .F. ) ;
#9216=CYLINDRICAL_SURFACE ( 'NONE', #4494, 1.699999999999996625 ) ;
#9219=CARTESIAN_POINT ( 'NONE',  ( 164.0000000000000568, 56.53993994372675047, 16.70000000000000995 ) ) ;
#9222=ORIENTED_EDGE ( 'NONE', *, *, #6089, .T. ) ;
#9224=CARTESIAN_POINT ( 'NONE',  ( 190.5000000000000568, 19.53993994372674692, -17.50000000000002487 ) ) ;
#9230=CIRCLE ( 'NONE', #14998, 3.500000000000003109 ) ;
#9231=FACE_OUTER_BOUND ( 'NONE', #14468, .T. ) ;
#9245=EDGE_CURVE ( 'NONE', #15197, #6193, #1777, .T. ) ;
#9250=VERTEX_POINT ( 'NONE', #12443 ) ;
#9262=VERTEX_POINT ( 'NONE', #276 ) ;
#9265=EDGE_LOOP ( 'NONE', ( #8558, #15248, #9213, #7440 ) ) ;
#9269=FACE_OUTER_BOUND ( 'NONE', #9, .T. ) ;
#9271=( NAMED_UNIT ( * ) SI_UNIT ( $, .STERADIAN. ) SOLID_ANGLE_UNIT ( ) );
#9283=DIRECTION ( 'NONE',  ( -0.000000000000000000, 1.000000000000000000, -0.000000000000000000 ) ) ;
#9288=ORIENTED_EDGE ( 'NONE', *, *, #10791, .F. ) ;
#9291=DIRECTION ( 'NONE',  ( 0.000000000000000000, -1.486905836551548832E-16, 1.000000000000000000 ) ) ;
#9292=CARTESIAN_POINT ( 'NONE',  ( -35.99999999999995026, 59.53993994372674337, 15.00000000000139977 ) ) ;
#9296=AXIS2_PLACEMENT_3D ( 'NONE', #12951, #15076, #2139 ) ;
#9297=VERTEX_POINT ( 'NONE', #11426 ) ;
#9298=ORIENTED_EDGE ( 'NONE', *, *, #9420, .T. ) ;
#9303=DIRECTION ( 'NONE',  ( 1.000000000000000000, 0.000000000000000000, 0.000000000000000000 ) ) ;
#9307=DIRECTION ( 'NONE',  ( 0.000000000000000000, 0.000000000000000000, -1.000000000000000000 ) ) ;
#9310=DIRECTION ( 'NONE',  ( -1.000000000000000000, 0.000000000000000000, 0.000000000000000000 ) ) ;
#9311=VECTOR ( 'NONE', #15019, 1000.000000000000000 ) ;
#9321=DIRECTION ( 'NONE',  ( 1.000000000000000000, 1.224646799147353207E-16, 1.062211776130383646E-32 ) ) ;
#9331=EDGE_CURVE ( 'NONE', #11744, #2137, #5263, .T. ) ;
#9340=ORIENTED_EDGE ( 'NONE', *, *, #1026, .F. ) ;
#9348=EDGE_CURVE ( 'NONE', #9928, #7532, #6337, .T. ) ;
#9362=CARTESIAN_POINT ( 'NONE',  ( 164.0000000000000568, 59.53993994372674337, 15.00000000000000355 ) ) ;
#9363=VECTOR ( 'NONE', #13139, 1000.000000000000000 ) ;
#9365=ORIENTED_EDGE ( 'NONE', *, *, #8034, .T. ) ;
#9368=DIRECTION ( 'NONE',  ( -0.000000000000000000, 1.000000000000000000, -0.000000000000000000 ) ) ;
#9372=CARTESIAN_POINT ( 'NONE',  ( -85.99999999999994316, 64.53993994372673626, 16.70000000000174012 ) ) ;
#9373=CARTESIAN_POINT ( 'NONE',  ( 224.0000000000000853, 19.53993994372674337, 9.999999999999998224 ) ) ;
#9375=DIRECTION ( 'NONE',  ( 0.000000000000000000, 0.000000000000000000, 1.000000000000000000 ) ) ;
#9382=DIRECTION ( 'NONE',  ( -0.000000000000000000, 1.000000000000000000, -0.000000000000000000 ) ) ;
#9393=DIRECTION ( 'NONE',  ( -0.000000000000000000, 1.000000000000000000, -0.000000000000000000 ) ) ;
#9396=FACE_BOUND ( 'NONE', #15470, .T. ) ;
#9397=CLOSED_SHELL ( 'NONE', ( #2856, #11280, #11985, #1364, #5786, #14528, #2574, #7127, #4217, #820, #7705, #5537, #7702, #11124, #13175, #984, #13287, #596, #9518, #9898, #3633, #7901, #10865, #12527, #10980, #13279, #2476, #14222, #10012, #83, #11446, #9503, #9752, #8180, #8274, #6245, #13596, #10774, #1151, #3565, #10991, #14602, #10640, #8323, #14840, #13070, #15013, #7785, #1220, #10469, #8887, #7464, #7750, #12699, #13583, #11676, #11358 ) ) ;
#9399=ADVANCED_FACE ( 'NONE', ( #8127 ), #2803, .F. ) ;
#9401=VERTEX_POINT ( 'NONE', #15036 ) ;
#9404=VERTEX_POINT ( 'NONE', #9219 ) ;
#9408=DIRECTION ( 'NONE',  ( 0.000000000000000000, 0.000000000000000000, 1.000000000000000000 ) ) ;
#9413=DIRECTION ( 'NONE',  ( 0.000000000000000000, 0.000000000000000000, -1.000000000000000000 ) ) ;
#9420=EDGE_CURVE ( 'NONE', #6168, #12024, #2024, .T. ) ;
#9422=VERTEX_POINT ( 'NONE', #7891 ) ;
#9424=EDGE_LOOP ( 'NONE', ( #12554, #5211 ) ) ;
#9427=CARTESIAN_POINT ( 'NONE',  ( 224.0000000000000853, 56.53993994372675047, 13.00000000000000178 ) ) ;
#9432=VECTOR ( 'NONE', #3986, 1000.000000000000000 ) ;
#9438=FACE_BOUND ( 'NONE', #14445, .T. ) ;
#9441=ORIENTED_EDGE ( 'NONE', *, *, #278, .F. ) ;
#9450=DIRECTION ( 'NONE',  ( -0.000000000000000000, 1.000000000000000000, -0.000000000000000000 ) ) ;
#9453=EDGE_CURVE ( 'NONE', #13487, #5951, #14092, .T. ) ;
#9468=CARTESIAN_POINT ( 'NONE',  ( 64.00000000000005684, 64.53993994372673626, 15.00000000000070166 ) ) ;
#9469=CARTESIAN_POINT ( 'NONE',  ( 14.00000000000004086, 64.51493994372674479, 18.50000000000105160 ) ) ;
#9475=DIRECTION ( 'NONE',  ( 1.000000000000000000, 0.000000000000000000, 0.000000000000000000 ) ) ;
#9487=CYLINDRICAL_SURFACE ( 'NONE', #6078, 3.500000000000003109 ) ;
#9501=VERTEX_POINT ( 'NONE', #14479 ) ;
#9502=DIRECTION ( 'NONE',  ( -0.000000000000000000, 1.000000000000000000, -0.000000000000000000 ) ) ;
#9503=ADVANCED_FACE ( 'NONE', ( #11895, #3674 ), #4700, .F. ) ;
#9511=LINE ( 'NONE', #7076, #1659 ) ;
#9518=ADVANCED_FACE ( 'NONE', ( #8356, #15579 ), #9763, .T. ) ;
#9524=DIRECTION ( 'NONE',  ( 0.000000000000000000, 1.486905836551548832E-16, -1.000000000000000000 ) ) ;
#9525=VERTEX_POINT ( 'NONE', #10633 ) ;
#9551=LINE ( 'NONE', #15239, #6313 ) ;
#9554=ORIENTED_EDGE ( 'NONE', *, *, #6815, .F. ) ;
#9555=VECTOR ( 'NONE', #3907, 1000.000000000000114 ) ;
#9556=EDGE_CURVE ( 'NONE', #12092, #10399, #1070, .T. ) ;
#9560=DIRECTION ( 'NONE',  ( 0.000000000000000000, 0.000000000000000000, 1.000000000000000000 ) ) ;
#9565=DIRECTION ( 'NONE',  ( 0.000000000000000000, -1.000000000000000000, 0.000000000000000000 ) ) ;
#9566=DIRECTION ( 'NONE',  ( 0.000000000000000000, -1.000000000000000000, -1.156482317317871478E-16 ) ) ;
#9568=VECTOR ( 'NONE', #8183, 1000.000000000000000 ) ;
#9571=EDGE_CURVE ( 'NONE', #3949, #12821, #9607, .T. ) ;
#9572=CARTESIAN_POINT ( 'NONE',  ( 114.0000000000000568, 62.13993994372673768, 15.00000000000035172 ) ) ;
#9574=CIRCLE ( 'NONE', #13334, 3.500000000000004885 ) ;
#9577=EDGE_LOOP ( 'NONE', ( #7120, #9106 ) ) ;
#9587=VERTEX_POINT ( 'NONE', #14404 ) ;
#9607=LINE ( 'NONE', #1300, #3308 ) ;
#9612=DIRECTION ( 'NONE',  ( 0.000000000000000000, -1.000000000000000000, 0.000000000000000000 ) ) ;
#9613=EDGE_CURVE ( 'NONE', #4660, #12466, #6133, .T. ) ;
#9614=CIRCLE ( 'NONE', #2541, 1.499999999999997780 ) ;
#9621=EDGE_CURVE ( 'NONE', #10088, #11744, #469, .T. ) ;
#9640=ORIENTED_EDGE ( 'NONE', *, *, #4702, .T. ) ;
#9649=DIRECTION ( 'NONE',  ( 0.000000000000000000, 0.000000000000000000, 1.000000000000000000 ) ) ;
#9656=ORIENTED_EDGE ( 'NONE', *, *, #9209, .T. ) ;
#9668=EDGE_LOOP ( 'NONE', ( #2550, #6111, #7755, #11063 ) ) ;
#9674=MECHANICAL_DESIGN_GEOMETRIC_PRESENTATION_REPRESENTATION('',(#13443),#2616);
#9675=ORIENTED_EDGE ( 'NONE', *, *, #9725, .F. ) ;
#9676=EDGE_CURVE ( 'NONE', #649, #3946, #4818, .T. ) ;
#9681=CIRCLE ( 'NONE', #3883, 1.499999999999997780 ) ;
#9686=DIRECTION ( 'NONE',  ( 0.000000000000000000, 8.673617379884035472E-17, -1.000000000000000000 ) ) ;
#9693=VECTOR ( 'NONE', #11820, 1000.000000000000000 ) ;
#9701=CARTESIAN_POINT ( 'NONE',  ( 185.1062858801516882, 25.86394065090268057, 18.00000000000000355 ) ) ;
#9705=ORIENTED_EDGE ( 'NONE', *, *, #15254, .F. ) ;
#9711=CARTESIAN_POINT ( 'NONE',  ( -35.99999999999995026, 64.53993994372673626, 15.00000000000139977 ) ) ;
#9712=DIRECTION ( 'NONE',  ( 0.000000000000000000, -1.000000000000000000, -1.156482317317871478E-16 ) ) ;
#9713=LINE ( 'NONE', #14503, #12511 ) ;
#9714=PLANE ( 'NONE',  #13857 ) ;
#9715=CARTESIAN_POINT ( 'NONE',  ( 14.00000000000004086, 62.13993994372673768, 15.00000000000104983 ) ) ;
#9720=ORIENTED_EDGE ( 'NONE', *, *, #4164, .T. ) ;
#9725=EDGE_CURVE ( 'NONE', #3061, #10088, #9028, .T. ) ;
#9729=AXIS2_PLACEMENT_3D ( 'NONE', #9199, #9040, #3113 ) ;
#9730=VERTEX_POINT ( 'NONE', #4428 ) ;
#9734=EDGE_LOOP ( 'NONE', ( #1134, #14535, #13491, #3711 ) ) ;
#9741=LINE ( 'NONE', #13432, #2244 ) ;
#9752=ADVANCED_FACE ( 'NONE', ( #2061, #12642, #14056 ), #10362, .T. ) ;
#9763=PLANE ( 'NONE',  #12627 ) ;
#9765=ORIENTED_EDGE ( 'NONE', *, *, #7417, .F. ) ;
#9771=EDGE_CURVE ( 'NONE', #11835, #10665, #7102, .T. ) ;
#9775=DIRECTION ( 'NONE',  ( 0.000000000000000000, 0.7071067811865474617, 0.7071067811865474617 ) ) ;
#9778=EDGE_CURVE ( 'NONE', #2210, #2673, #6348, .T. ) ;
#9781=CARTESIAN_POINT ( 'NONE',  ( 64.00000000000005684, 64.53993994372673626, 18.52500000000070202 ) ) ;
#9786=DIRECTION ( 'NONE',  ( 0.000000000000000000, 0.000000000000000000, -1.000000000000000000 ) ) ;
#9798=DIRECTION ( 'NONE',  ( -0.000000000000000000, 1.000000000000000000, -0.000000000000000000 ) ) ;
#9803=LINE ( 'NONE', #14601, #15128 ) ;
#9805=EDGE_CURVE ( 'NONE', #2217, #14095, #12380, .T. ) ;
#9807=DIRECTION ( 'NONE',  ( -0.000000000000000000, 1.000000000000000000, -0.000000000000000000 ) ) ;
#9809=EDGE_CURVE ( 'NONE', #6601, #163, #7612, .T. ) ;
#9813=DIRECTION ( 'NONE',  ( 0.000000000000000000, 0.000000000000000000, 1.000000000000000000 ) ) ;
#9820=DIRECTION ( 'NONE',  ( -0.000000000000000000, 1.000000000000000000, -0.000000000000000000 ) ) ;
#9821=CARTESIAN_POINT ( 'NONE',  ( -76.50000000000001421, 17.53993994372674692, -17.50000000000002487 ) ) ;
#9823=EDGE_LOOP ( 'NONE', ( #13196, #15427 ) ) ;
#9828=CARTESIAN_POINT ( 'NONE',  ( -110.0000000000000426, 19.53993994372674337, 9.999999999999998224 ) ) ;
#9831=VECTOR ( 'NONE', #162, 1000.000000000000114 ) ;
#9835=ORIENTED_EDGE ( 'NONE', *, *, #5254, .F. ) ;
#9838=VERTEX_POINT ( 'NONE', #7050 ) ;
#9848=VECTOR ( 'NONE', #12490, 1000.000000000000000 ) ;
#9863=CARTESIAN_POINT ( 'NONE',  ( -110.0000000000000426, 56.53993994372675047, 25.00000000000000000 ) ) ;
#9868=CARTESIAN_POINT ( 'NONE',  ( -110.0000000000000426, 22.53993994372673981, 24.99999999999999645 ) ) ;
#9875=ORIENTED_EDGE ( 'NONE', *, *, #9331, .F. ) ;
#9883=EDGE_LOOP ( 'NONE', ( #12907, #12555 ) ) ;
#9892=LINE ( 'NONE', #5295, #11170 ) ;
#9898=ADVANCED_FACE ( 'NONE', ( #11781 ), #4741, .T. ) ;
#9905=EDGE_CURVE ( 'NONE', #15478, #8543, #14367, .T. ) ;
#9909=EDGE_CURVE ( 'NONE', #9404, #2275, #11652, .T. ) ;
#9910=AXIS2_PLACEMENT_3D ( 'NONE', #1580, #6416, #7445 ) ;
#9912=CARTESIAN_POINT ( 'NONE',  ( -85.99999999999994316, 64.53993994372673626, 13.30000000000175575 ) ) ;
#9920=ORIENTED_EDGE ( 'NONE', *, *, #625, .T. ) ;
#9928=VERTEX_POINT ( 'NONE', #10836 ) ;
#9932=LINE ( 'NONE', #12277, #9432 ) ;
#9933=FACE_OUTER_BOUND ( 'NONE', #8242, .T. ) ;
#9941=ORIENTED_EDGE ( 'NONE', *, *, #10593, .T. ) ;
#9944=CARTESIAN_POINT ( 'NONE',  ( -35.99999999999995026, 64.53993994372673626, 18.52500000000140190 ) ) ;
#9945=FACE_OUTER_BOUND ( 'NONE', #2613, .T. ) ;
#9947=CARTESIAN_POINT ( 'NONE',  ( -76.50000000000001421, 19.53993994372674692, -17.50000000000002487 ) ) ;
#9956=EDGE_CURVE ( 'NONE', #9422, #13622, #10035, .T. ) ;
#9960=VERTEX_POINT ( 'NONE', #1338 ) ;
#9966=CARTESIAN_POINT ( 'NONE',  ( 215.1062858801516882, 25.86394065090268057, 18.00000000000000355 ) ) ;
#9967=FACE_OUTER_BOUND ( 'NONE', #4681, .T. ) ;
#9968=AXIS2_PLACEMENT_3D ( 'NONE', #819, #13861, #13940 ) ;
#9971=ORIENTED_EDGE ( 'NONE', *, *, #3662, .T. ) ;
#9977=VERTEX_POINT ( 'NONE', #8769 ) ;
#9982=ORIENTED_EDGE ( 'NONE', *, *, #8786, .T. ) ;
#9986=VERTEX_POINT ( 'NONE', #6411 ) ;
#9987=CYLINDRICAL_SURFACE ( 'NONE', #13593, 3.500000000000003109 ) ;
#10000=ORIENTED_EDGE ( 'NONE', *, *, #9771, .T. ) ;
#10005=TOROIDAL_SURFACE ( 'NONE', #5711, 6.999999999999991118, 2.000000000000000000 ) ;
#10011=EDGE_CURVE ( 'NONE', #10092, #5037, #1654, .T. ) ;
#10012=ADVANCED_FACE ( 'NONE', ( #5451 ), #11288, .F. ) ;
#10013=VECTOR ( 'NONE', #8459, 1000.000000000000000 ) ;
#10019=VERTEX_POINT ( 'NONE', #449 ) ;
#10020=EDGE_LOOP ( 'NONE', ( #11929, #1009, #4511, #6911 ) ) ;
#10023=CARTESIAN_POINT ( 'NONE',  ( 164.0000000000000568, 62.13993994372673768, 11.50000000000000000 ) ) ;
#10024=DIRECTION ( 'NONE',  ( -0.000000000000000000, 1.000000000000000000, -0.000000000000000000 ) ) ;
#10033=ORIENTED_EDGE ( 'NONE', *, *, #4815, .F. ) ;
#10035=LINE ( 'NONE', #2693, #29 ) ;
#10037=DIRECTION ( 'NONE',  ( -1.000000000000000000, 0.000000000000000000, -0.000000000000000000 ) ) ;
#10038=CARTESIAN_POINT ( 'NONE',  ( -35.99999999999995026, 62.13993994372673768, 15.00000000000139977 ) ) ;
#10039=EDGE_CURVE ( 'NONE', #8632, #8731, #14980, .T. ) ;
#10044=ORIENTED_EDGE ( 'NONE', *, *, #9119, .F. ) ;
#10045=DIRECTION ( 'NONE',  ( -0.000000000000000000, 1.000000000000000000, 8.673617379884035472E-17 ) ) ;
#10047=ORIENTED_EDGE ( 'NONE', *, *, #4211, .T. ) ;
#10057=FACE_BOUND ( 'NONE', #8767, .T. ) ;
#10062=CIRCLE ( 'NONE', #14336, 1.699999999999993072 ) ;
#10066=FACE_BOUND ( 'NONE', #6000, .T. ) ;
#10067=DIRECTION ( 'NONE',  ( 0.000000000000000000, 0.000000000000000000, 1.000000000000000000 ) ) ;
#10076=EDGE_CURVE ( 'NONE', #9198, #13912, #2823, .T. ) ;
#10079=AXIS2_PLACEMENT_3D ( 'NONE', #6673, #5478, #1832 ) ;
#10081=DIRECTION ( 'NONE',  ( 0.000000000000000000, 0.000000000000000000, 1.000000000000000000 ) ) ;
#10087=DIRECTION ( 'NONE',  ( 0.000000000000000000, 0.000000000000000000, 1.000000000000000000 ) ) ;
#10088=VERTEX_POINT ( 'NONE', #12623 ) ;
#10092=VERTEX_POINT ( 'NONE', #10420 ) ;
#10093=CIRCLE ( 'NONE', #233, 3.524999999999998579 ) ;
#10094=DIRECTION ( 'NONE',  ( -1.000000000000000000, -4.585547486636276518E-32, 3.965082230804130220E-16 ) ) ;
#10097=CARTESIAN_POINT ( 'NONE',  ( 164.0000000000000568, 62.13993994372673768, 15.00000000000000355 ) ) ;
#10106=AXIS2_PLACEMENT_3D ( 'NONE', #4295, #5651, #11657 ) ;
#10111=ORIENTED_EDGE ( 'NONE', *, *, #1114, .T. ) ;
#10115=EDGE_LOOP ( 'NONE', ( #7281, #7920 ) ) ;
#10119=AXIS2_PLACEMENT_3D ( 'NONE', #7567, #12366, #348 ) ;
#10128=CIRCLE ( 'NONE', #521, 1.699999999999991518 ) ;
#10131=ORIENTED_EDGE ( 'NONE', *, *, #2880, .T. ) ;
#10135=DIRECTION ( 'NONE',  ( -0.000000000000000000, -0.000000000000000000, 1.000000000000000000 ) ) ;
#10137=DIRECTION ( 'NONE',  ( 0.000000000000000000, 0.000000000000000000, 1.000000000000000000 ) ) ;
#10144=ADVANCED_FACE ( 'NONE', ( #12695, #4330 ), #11373, .F. ) ;
#10162=CARTESIAN_POINT ( 'NONE',  ( 185.1062858801516882, 25.86394065090268057, 18.00000000000000355 ) ) ;
#10165=FACE_OUTER_BOUND ( 'NONE', #6548, .T. ) ;
#10167=EDGE_LOOP ( 'NONE', ( #7238, #293 ) ) ;
#10169=CARTESIAN_POINT ( 'NONE',  ( 184.0000000000000568, 19.53993994372673626, 47.49999999999997868 ) ) ;
#10171=ORIENTED_EDGE ( 'NONE', *, *, #9613, .F. ) ;
#10173=DIRECTION ( 'NONE',  ( 8.659560562355533132E-17, 0.7071067811864985009, -0.7071067811865965336 ) ) ;
#10177=CIRCLE ( 'NONE', #1585, 4.999999999999990230 ) ;
#10180=PLANE ( 'NONE',  #3124 ) ;
#10188=ORIENTED_EDGE ( 'NONE', *, *, #12399, .T. ) ;
#10190=CARTESIAN_POINT ( 'NONE',  ( -84.29999999999994031, 62.13993994372673768, 15.00000000000174794 ) ) ;
#10196=CARTESIAN_POINT ( 'NONE',  ( 164.0000000000000568, 62.13993994372673768, 18.50000000000000711 ) ) ;
#10197=VERTEX_POINT ( 'NONE', #8065 ) ;
#10217=CARTESIAN_POINT ( 'NONE',  ( 165.7000000000000739, 62.13993994372673768, 15.00000000000000355 ) ) ;
#10234=LINE ( 'NONE', #3051, #2026 ) ;
#10241=CARTESIAN_POINT ( 'NONE',  ( 114.0000000000000568, 64.53993994372673626, 15.00000000000035172 ) ) ;
#10243=VERTEX_POINT ( 'NONE', #15370 ) ;
#10245=VERTEX_POINT ( 'NONE', #7033 ) ;
#10247=FACE_OUTER_BOUND ( 'NONE', #12691, .T. ) ;
#10249=DIRECTION ( 'NONE',  ( -0.000000000000000000, 1.000000000000000000, 1.156482317317871725E-16 ) ) ;
#10256=DIRECTION ( 'NONE',  ( 0.000000000000000000, 0.000000000000000000, 1.000000000000000000 ) ) ;
#10257=EDGE_CURVE ( 'NONE', #13079, #12092, #7117, .T. ) ;
#10263=ORIENTED_EDGE ( 'NONE', *, *, #9109, .F. ) ;
#10265=DIRECTION ( 'NONE',  ( 0.000000000000000000, -1.000000000000000000, 0.000000000000000000 ) ) ;
#10268=CARTESIAN_POINT ( 'NONE',  ( 64.00000000000005684, 64.53993994372673626, 13.30000000000070948 ) ) ;
#10271=EDGE_LOOP ( 'NONE', ( #14189, #8227, #3406, #958 ) ) ;
#10282=EDGE_CURVE ( 'NONE', #2947, #11184, #5684, .T. ) ;
#10283=CARTESIAN_POINT ( 'NONE',  ( -85.99999999999994316, 59.53993994372674337, 15.00000000000174794 ) ) ;
#10285=VECTOR ( 'NONE', #5836, 1000.000000000000000 ) ;
#10289=CARTESIAN_POINT ( 'NONE',  ( 64.00000000000005684, 64.53993994372673626, 15.00000000000070166 ) ) ;
#10299=CARTESIAN_POINT ( 'NONE',  ( 114.0000000000000568, 64.53993994372673626, 15.00000000000035172 ) ) ;
#10300=AXIS2_PLACEMENT_3D ( 'NONE', #1461, #1317, #6300 ) ;
#10303=VERTEX_POINT ( 'NONE', #12933 ) ;
#10307=EDGE_CURVE ( 'NONE', #899, #8731, #10128, .T. ) ;
#10313=CARTESIAN_POINT ( 'NONE',  ( 114.0000000000000568, 56.53993994372675047, 15.00000000000035172 ) ) ;
#10315=EDGE_LOOP ( 'NONE', ( #8826, #4822 ) ) ;
#10318=DIRECTION ( 'NONE',  ( -0.000000000000000000, 1.000000000000000000, -0.000000000000000000 ) ) ;
#10319=AXIS2_PLACEMENT_3D ( 'NONE', #2850, #2614, #6330 ) ;
#10329=CARTESIAN_POINT ( 'NONE',  ( 185.1062858801516882, 25.86394065090268057, 18.00000000000000355 ) ) ;
#10332=DIRECTION ( 'NONE',  ( 0.000000000000000000, 1.000000000000000000, 0.000000000000000000 ) ) ;
#10333=DIRECTION ( 'NONE',  ( 1.000000000000000000, 0.000000000000000000, 0.000000000000000000 ) ) ;
#10334=DIRECTION ( 'NONE',  ( 0.000000000000000000, -1.000000000000000000, -1.156482317317871478E-16 ) ) ;
#10345=CARTESIAN_POINT ( 'NONE',  ( 185.1062858801516882, 25.86394065090268057, 18.00000000000000355 ) ) ;
#10347=DIRECTION ( 'NONE',  ( 0.000000000000000000, 0.000000000000000000, 1.000000000000000000 ) ) ;
#10350=ORIENTED_EDGE ( 'NONE', *, *, #10257, .F. ) ;
#10358=AXIS2_PLACEMENT_3D ( 'NONE', #5455, #12936, #15141 ) ;
#10362=PLANE ( 'NONE',  #13126 ) ;
#10369=DIRECTION ( 'NONE',  ( -0.000000000000000000, -0.000000000000000000, 1.000000000000000000 ) ) ;
#10373=AXIS2_PLACEMENT_3D ( 'NONE', #11176, #327, #5167 ) ;
#10378=CARTESIAN_POINT ( 'NONE',  ( 207.1062858801516597, 40.86394065090267702, 18.00000000000001066 ) ) ;
#10379=VERTEX_POINT ( 'NONE', #12066 ) ;
#10382=VERTEX_POINT ( 'NONE', #9781 ) ;
#10383=AXIS2_PLACEMENT_3D ( 'NONE', #15391, #5775, #7286 ) ;
#10392=EDGE_CURVE ( 'NONE', #10665, #11835, #10632, .T. ) ;
#10399=VERTEX_POINT ( 'NONE', #13316 ) ;
#10403=DIRECTION ( 'NONE',  ( 0.000000000000000000, 0.000000000000000000, 1.000000000000000000 ) ) ;
#10404=LINE ( 'NONE', #9224, #14800 ) ;
#10405=CARTESIAN_POINT ( 'NONE',  ( 185.1062858801516882, 25.86394065090268057, 13.00000000000000178 ) ) ;
#10412=DIRECTION ( 'NONE',  ( 0.000000000000000000, -1.000000000000000000, -1.156482317317871478E-16 ) ) ;
#10415=CARTESIAN_POINT ( 'NONE',  ( 114.0000000000000568, 64.53993994372673626, 15.00000000000035172 ) ) ;
#10420=CARTESIAN_POINT ( 'NONE',  ( 177.5000000000000853, 19.53993994372673626, 52.49999999999997868 ) ) ;
#10422=ORIENTED_EDGE ( 'NONE', *, *, #4891, .F. ) ;
#10437=VERTEX_POINT ( 'NONE', #6310 ) ;
#10441=ORIENTED_EDGE ( 'NONE', *, *, #7642, .T. ) ;
#10445=ORIENTED_EDGE ( 'NONE', *, *, #8690, .T. ) ;
#10447=CIRCLE ( 'NONE', #8188, 1.499999999999997780 ) ;
#10465=CARTESIAN_POINT ( 'NONE',  ( -35.99999999999995026, 62.13993994372673768, 16.70000000000140261 ) ) ;
#10467=DIRECTION ( 'NONE',  ( 0.000000000000000000, 0.000000000000000000, 1.000000000000000000 ) ) ;
#10469=ADVANCED_FACE ( 'NONE', ( #9945 ), #6925, .F. ) ;
#10470=ORIENTED_EDGE ( 'NONE', *, *, #10282, .F. ) ;
#10473=ORIENTED_EDGE ( 'NONE', *, *, #8276, .F. ) ;
#10481=ORIENTED_EDGE ( 'NONE', *, *, #10773, .T. ) ;
#10483=DIRECTION ( 'NONE',  ( 3.965082230804130220E-16, -1.486905836551548832E-16, 1.000000000000000000 ) ) ;
#10491=CARTESIAN_POINT ( 'NONE',  ( -110.0000000000000426, 19.53993994372674337, 9.999999999999998224 ) ) ;
#10497=EDGE_LOOP ( 'NONE', ( #6192, #13707, #15419, #12267 ) ) ;
#10506=ORIENTED_EDGE ( 'NONE', *, *, #5254, .T. ) ;
#10508=EDGE_CURVE ( 'NONE', #10243, #9525, #14974, .T. ) ;
#10520=AXIS2_PLACEMENT_3D ( 'NONE', #14965, #13632, #11354 ) ;
#10523=ORIENTED_EDGE ( 'NONE', *, *, #1251, .F. ) ;
#10527=ORIENTED_EDGE ( 'NONE', *, *, #2163, .F. ) ;
#10529=UNCERTAINTY_MEASURE_WITH_UNIT (LENGTH_MEASURE( 1.000000000000000082E-05 ), #15547, 'distance_accuracy_value', 'NONE');
#10535=DIRECTION ( 'NONE',  ( 1.000000000000000000, -0.000000000000000000, -0.000000000000000000 ) ) ;
#10538=EDGE_LOOP ( 'NONE', ( #7523, #8189, #11424, #12397 ) ) ;
#10547=LINE ( 'NONE', #13297, #5554 ) ;
#10553=LINE ( 'NONE', #4312, #9693 ) ;
#10554=FACE_OUTER_BOUND ( 'NONE', #12703, .T. ) ;
#10557=DIRECTION ( 'NONE',  ( -0.000000000000000000, 1.000000000000000000, -0.000000000000000000 ) ) ;
#10561=DIRECTION ( 'NONE',  ( 0.000000000000000000, 0.000000000000000000, -1.000000000000000000 ) ) ;
#10562=AXIS2_PLACEMENT_3D ( 'NONE', #15600, #5993, #14422 ) ;
#10565=AXIS2_PLACEMENT_3D ( 'NONE', #5578, #9283, #10467 ) ;
#10570=DIRECTION ( 'NONE',  ( -0.000000000000000000, 1.000000000000000000, 1.156482317317871725E-16 ) ) ;
#10575=ORIENTED_EDGE ( 'NONE', *, *, #14000, .T. ) ;
#10578=VERTEX_POINT ( 'NONE', #4297 ) ;
#10586=VERTEX_POINT ( 'NONE', #497 ) ;
#10587=AXIS2_PLACEMENT_3D ( 'NONE', #10289, #13916, #3107 ) ;
#10593=EDGE_CURVE ( 'NONE', #6121, #10896, #8119, .T. ) ;
#10595=ADVANCED_FACE ( 'NONE', ( #11416 ), #7956, .F. ) ;
#10610=ORIENTED_EDGE ( 'NONE', *, *, #6218, .T. ) ;
#10612=CIRCLE ( 'NONE', #15130, 3.500000000000003109 ) ;
#10621=CARTESIAN_POINT ( 'NONE',  ( 184.0000000000000568, 17.53993994372673271, 45.99999999999998579 ) ) ;
#10623=EDGE_CURVE ( 'NONE', #973, #5616, #6619, .T. ) ;
#10626=CARTESIAN_POINT ( 'NONE',  ( -85.99999999999994316, 64.53993994372673626, 15.00000000000174794 ) ) ;
#10631=CARTESIAN_POINT ( 'NONE',  ( 114.0000000000000568, 64.53993994372673626, 15.00000000000035172 ) ) ;
#10632=CIRCLE ( 'NONE', #12637, 5.000000000000004441 ) ;
#10633=CARTESIAN_POINT ( 'NONE',  ( -85.99999999999994316, 59.53993994372674337, 13.30000000000175575 ) ) ;
#10635=VERTEX_POINT ( 'NONE', #4454 ) ;
#10640=ADVANCED_FACE ( 'NONE', ( #4218, #8982 ), #9056, .T. ) ;
#10646=AXIS2_PLACEMENT_3D ( 'NONE', #8145, #12848, #4718 ) ;
#10648=LINE ( 'NONE', #15438, #12963 ) ;
#10659=DIRECTION ( 'NONE',  ( -0.000000000000000000, 1.000000000000000000, -0.000000000000000000 ) ) ;
#10662=AXIS2_PLACEMENT_3D ( 'NONE', #2203, #10659, #15447 ) ;
#10665=VERTEX_POINT ( 'NONE', #5420 ) ;
#10668=AXIS2_PLACEMENT_3D ( 'NONE', #4082, #5196, #280 ) ;
#10670=LINE ( 'NONE', #5769, #2481 ) ;
#10675=DIRECTION ( 'NONE',  ( -0.000000000000000000, 1.486905836551548832E-16, -1.000000000000000000 ) ) ;
#10686=VECTOR ( 'NONE', #12375, 1000.000000000000000 ) ;
#10687=DIRECTION ( 'NONE',  ( 1.000000000000000000, 0.000000000000000000, 0.000000000000000000 ) ) ;
#10695=AXIS2_PLACEMENT_3D ( 'NONE', #1457, #267, #13534 ) ;
#10709=DIRECTION ( 'NONE',  ( 0.000000000000000000, 0.000000000000000000, 1.000000000000000000 ) ) ;
#10710=CARTESIAN_POINT ( 'NONE',  ( 114.0000000000000568, 64.53993994372673626, 13.30000000000035776 ) ) ;
#10718=DIRECTION ( 'NONE',  ( -1.000000000000000000, 0.000000000000000000, 0.000000000000000000 ) ) ;
#10721=DIRECTION ( 'NONE',  ( 1.000000000000000000, 0.000000000000000000, 0.000000000000000000 ) ) ;
#10729=ORIENTED_EDGE ( 'NONE', *, *, #5051, .F. ) ;
#10735=LINE ( 'NONE', #126, #11024 ) ;
#10737=DIRECTION ( 'NONE',  ( -1.000000000000000000, 0.000000000000000000, 0.000000000000000000 ) ) ;
#10739=CIRCLE ( 'NONE', #5439, 1.699999999999993072 ) ;
#10742=VERTEX_POINT ( 'NONE', #14162 ) ;
#10756=ORIENTED_EDGE ( 'NONE', *, *, #10307, .T. ) ;
#10757=CARTESIAN_POINT ( 'NONE',  ( 195.1062858801516597, 40.86394065090267702, 12.00000000000001066 ) ) ;
#10769=ORIENTED_EDGE ( 'NONE', *, *, #10806, .T. ) ;
#10773=EDGE_CURVE ( 'NONE', #8016, #2806, #2718, .T. ) ;
#10774=ADVANCED_FACE ( 'NONE', ( #324 ), #2805, .F. ) ;
#10779=CARTESIAN_POINT ( 'NONE',  ( 114.0000000000000568, 62.13993994372673768, 15.00000000000035172 ) ) ;
#10785=CARTESIAN_POINT ( 'NONE',  ( 185.1062858801516882, 55.86394065090267702, 13.00000000000000178 ) ) ;
#10791=EDGE_CURVE ( 'NONE', #10635, #3817, #4594, .T. ) ;
#10792=ORIENTED_EDGE ( 'NONE', *, *, #7608, .F. ) ;
#10795=ORIENTED_EDGE ( 'NONE', *, *, #11550, .T. ) ;
#10796=CARTESIAN_POINT ( 'NONE',  ( 64.00000000000005684, 59.53993994372674337, 16.70000000000069562 ) ) ;
#10797=PLANE ( 'NONE',  #11335 ) ;
#10798=VECTOR ( 'NONE', #10993, 1000.000000000000000 ) ;
#10799=FACE_OUTER_BOUND ( 'NONE', #9734, .T. ) ;
#10806=EDGE_CURVE ( 'NONE', #649, #3817, #8649, .T. ) ;
#10808=DIRECTION ( 'NONE',  ( 0.000000000000000000, -1.000000000000000000, -1.156482317317871478E-16 ) ) ;
#10809=CARTESIAN_POINT ( 'NONE',  ( 185.1062858801516882, 55.86394065090267702, 13.00000000000000178 ) ) ;
#10817=FACE_OUTER_BOUND ( 'NONE', #7378, .T. ) ;
#10820=DIRECTION ( 'NONE',  ( 0.000000000000000000, -1.000000000000000000, -1.156482317317871478E-16 ) ) ;
#10833=EDGE_LOOP ( 'NONE', ( #6020, #9130, #778, #12230 ) ) ;
#10834=ORIENTED_EDGE ( 'NONE', *, *, #6731, .T. ) ;
#10836=CARTESIAN_POINT ( 'NONE',  ( 64.00000000000005684, 59.53993994372674337, 13.30000000000070948 ) ) ;
#10838=VECTOR ( 'NONE', #1429, 1000.000000000000000 ) ;
#10842=AXIS2_PLACEMENT_3D ( 'NONE', #5586, #3130, #10087 ) ;
#10843=CARTESIAN_POINT ( 'NONE',  ( -110.0000000000000426, 19.53993994372674337, 24.99999999999999645 ) ) ;
#10852=VECTOR ( 'NONE', #5426, 1000.000000000000000 ) ;
#10854=ORIENTED_EDGE ( 'NONE', *, *, #6610, .F. ) ;
#10857=VECTOR ( 'NONE', #6594, 1000.000000000000000 ) ;
#10859=LINE ( 'NONE', #13038, #3766 ) ;
#10860=FACE_BOUND ( 'NONE', #7295, .T. ) ;
#10865=ADVANCED_FACE ( 'NONE', ( #2644, #7465, #12259, #1526, #6362, #12801, #7707 ), #15243, .T. ) ;
#10868=EDGE_LOOP ( 'NONE', ( #14082, #13975, #12953, #8480 ) ) ;
#10870=CARTESIAN_POINT ( 'NONE',  ( -110.0000000000000426, 19.53993994372674337, 9.999999999999998224 ) ) ;
#10873=ORIENTED_EDGE ( 'NONE', *, *, #1736, .F. ) ;
#10877=ORIENTED_EDGE ( 'NONE', *, *, #14236, .F. ) ;
#10889=FACE_OUTER_BOUND ( 'NONE', #7174, .T. ) ;
#10892=LINE ( 'NONE', #11117, #12300 ) ;
#10896=VERTEX_POINT ( 'NONE', #15167 ) ;
#10899=CYLINDRICAL_SURFACE ( 'NONE', #2840, 1.700000000000001954 ) ;
#10902=FACE_OUTER_BOUND ( 'NONE', #12080, .T. ) ;
#10904=ADVANCED_FACE ( 'NONE', ( #4438 ), #1837, .F. ) ;
#10910=ORIENTED_EDGE ( 'NONE', *, *, #3279, .F. ) ;
#10913=ORIENTED_EDGE ( 'NONE', *, *, #11149, .T. ) ;
#10915=CIRCLE ( 'NONE', #5866, 1.700000000000007061 ) ;
#10917=ORIENTED_EDGE ( 'NONE', *, *, #15166, .F. ) ;
#10938=DIRECTION ( 'NONE',  ( 0.000000000000000000, 1.000000000000000000, 0.000000000000000000 ) ) ;
#10940=ORIENTED_EDGE ( 'NONE', *, *, #12915, .T. ) ;
#10942=DIRECTION ( 'NONE',  ( 0.000000000000000000, -1.000000000000000000, -1.156482317317871725E-16 ) ) ;
#10947=AXIS2_PLACEMENT_3D ( 'NONE', #8669, #2588, #10081 ) ;
#10951=ORIENTED_EDGE ( 'NONE', *, *, #9909, .F. ) ;
#10953=DIRECTION ( 'NONE',  ( 8.659560562354932858E-17, 0.7071067811865474617, -0.7071067811865474617 ) ) ;
#10957=DIRECTION ( 'NONE',  ( 0.000000000000000000, 0.000000000000000000, 1.000000000000000000 ) ) ;
#10958=EDGE_CURVE ( 'NONE', #4614, #12779, #13994, .T. ) ;
#10959=DIRECTION ( 'NONE',  ( 0.000000000000000000, 0.000000000000000000, 1.000000000000000000 ) ) ;
#10965=DIRECTION ( 'NONE',  ( -0.000000000000000000, 1.000000000000000000, -0.000000000000000000 ) ) ;
#10974=FACE_BOUND ( 'NONE', #8551, .T. ) ;
#10976=EDGE_CURVE ( 'NONE', #5209, #13055, #3111, .T. ) ;
#10977=EDGE_CURVE ( 'NONE', #13329, #11305, #4527, .T. ) ;
#10980=ADVANCED_FACE ( 'NONE', ( #13759 ), #1761, .T. ) ;
#10981=ORIENTED_EDGE ( 'NONE', *, *, #15191, .F. ) ;
#10982=ORIENTED_EDGE ( 'NONE', *, *, #9453, .F. ) ;
#10990=CIRCLE ( 'NONE', #4945, 1.700000000000000178 ) ;
#10991=ADVANCED_FACE ( 'NONE', ( #4278, #8178 ), #11946, .T. ) ;
#10993=DIRECTION ( 'NONE',  ( -0.000000000000000000, 1.000000000000000000, 1.156482317317871725E-16 ) ) ;
#10997=ORIENTED_EDGE ( 'NONE', *, *, #12547, .F. ) ;
#10998=EDGE_LOOP ( 'NONE', ( #11429, #8932, #8853, #15528 ) ) ;
#11004=EDGE_LOOP ( 'NONE', ( #9656, #1 ) ) ;
#11011=AXIS2_PLACEMENT_3D ( 'NONE', #14582, #7273, #15527 ) ;
#11024=VECTOR ( 'NONE', #8382, 1000.000000000000000 ) ;
#11036=ORIENTED_EDGE ( 'NONE', *, *, #6650, .T. ) ;
#11041=LINE ( 'NONE', #9868, #692 ) ;
#11047=LINE ( 'NONE', #2522, #15354 ) ;
#11051=VECTOR ( 'NONE', #10173, 1000.000000000000000 ) ;
#11052=DIRECTION ( 'NONE',  ( 0.000000000000000000, 0.000000000000000000, -1.000000000000000000 ) ) ;
#11057=EDGE_CURVE ( 'NONE', #4694, #3509, #11869, .T. ) ;
#11063=ORIENTED_EDGE ( 'NONE', *, *, #13225, .T. ) ;
#11068=DIRECTION ( 'NONE',  ( 3.965082230804130220E-16, 1.486905836551548832E-16, -1.000000000000000000 ) ) ;
#11070=MANIFOLD_SOLID_BREP ( 'Fillet4', #9397 ) ;
#11073=ADVANCED_FACE ( 'NONE', ( #8101 ), #12886, .F. ) ;
#11075=EDGE_CURVE ( 'NONE', #15428, #899, #12245, .T. ) ;
#11077=ORIENTED_EDGE ( 'NONE', *, *, #4140, .F. ) ;
#11087=LINE ( 'NONE', #2639, #11496 ) ;
#11091=EDGE_CURVE ( 'NONE', #12980, #1879, #5071, .T. ) ;
#11097=FACE_OUTER_BOUND ( 'NONE', #7131, .T. ) ;
#11098=VECTOR ( 'NONE', #6259, 1000.000000000000000 ) ;
#11110=DIRECTION ( 'NONE',  ( 0.000000000000000000, 0.000000000000000000, 1.000000000000000000 ) ) ;
#11111=EDGE_CURVE ( 'NONE', #627, #9960, #13206, .T. ) ;
#11117=CARTESIAN_POINT ( 'NONE',  ( -76.50000000000004263, 17.53993994372673271, 52.49999999999997868 ) ) ;
#11122=CARTESIAN_POINT ( 'NONE',  ( 14.00000000000004086, 59.53993994372674337, 13.30000000000105231 ) ) ;
#11124=ADVANCED_FACE ( 'NONE', ( #8482 ), #14610, .T. ) ;
#11125=EDGE_LOOP ( 'NONE', ( #12753, #2919, #1570, #3205 ) ) ;
#11127=DIRECTION ( 'NONE',  ( -0.000000000000000000, 1.000000000000000000, 1.156482317317871725E-16 ) ) ;
#11129=DIRECTION ( 'NONE',  ( 0.000000000000000000, 0.000000000000000000, 1.000000000000000000 ) ) ;
#11134=AXIS2_PLACEMENT_3D ( 'NONE', #2492, #2414, #9524 ) ;
#11141=ORIENTED_EDGE ( 'NONE', *, *, #9778, .F. ) ;
#11147=CYLINDRICAL_SURFACE ( 'NONE', #6587, 1.699999999999991518 ) ;
#11149=EDGE_CURVE ( 'NONE', #299, #14837, #2627, .T. ) ;
#11151=VERTEX_POINT ( 'NONE', #6423 ) ;
#11154=FACE_OUTER_BOUND ( 'NONE', #8184, .T. ) ;
#11155=CIRCLE ( 'NONE', #8401, 3.500000000000004885 ) ;
#11168=ADVANCED_FACE ( 'NONE', ( #11154 ), #1425, .F. ) ;
#11170=VECTOR ( 'NONE', #13422, 1000.000000000000000 ) ;
#11176=CARTESIAN_POINT ( 'NONE',  ( -110.0000000000000426, 59.53993994372674337, 25.00000000000000000 ) ) ;
#11180=ORIENTED_EDGE ( 'NONE', *, *, #11550, .F. ) ;
#11182=CIRCLE ( 'NONE', #4609, 1.699999999999998401 ) ;
#11184=VERTEX_POINT ( 'NONE', #2460 ) ;
#11187=DIRECTION ( 'NONE',  ( 0.000000000000000000, 0.000000000000000000, 1.000000000000000000 ) ) ;
#11193=CARTESIAN_POINT ( 'NONE',  ( -85.99999999999994316, 62.13993994372673768, 15.00000000000174794 ) ) ;
#11194=DIRECTION ( 'NONE',  ( -0.000000000000000000, 1.000000000000000000, 0.000000000000000000 ) ) ;
#11195=ORIENTED_EDGE ( 'NONE', *, *, #4899, .F. ) ;
#11198=ORIENTED_EDGE ( 'NONE', *, *, #7608, .T. ) ;
#11199=EDGE_LOOP ( 'NONE', ( #5338, #10769, #3208, #11286 ) ) ;
#11203=FACE_BOUND ( 'NONE', #10315, .T. ) ;
#11227=VERTEX_POINT ( 'NONE', #4562 ) ;
#11234=ORIENTED_EDGE ( 'NONE', *, *, #6146, .T. ) ;
#11240=DIRECTION ( 'NONE',  ( 0.000000000000000000, 0.000000000000000000, 1.000000000000000000 ) ) ;
#11252=EDGE_CURVE ( 'NONE', #11722, #1879, #14106, .T. ) ;
#11253=ORIENTED_EDGE ( 'NONE', *, *, #1398, .T. ) ;
#11258=VECTOR ( 'NONE', #1985, 1000.000000000000000 ) ;
#11260=CARTESIAN_POINT ( 'NONE',  ( -110.0000000000000426, 56.53993994372675047, 25.00000000000000000 ) ) ;
#11272=DIRECTION ( 'NONE',  ( 0.000000000000000000, -1.000000000000000000, -1.156482317317871478E-16 ) ) ;
#11277=CARTESIAN_POINT ( 'NONE',  ( 114.0000000000000568, 62.13993994372673768, 11.50000000000034817 ) ) ;
#11279=ORIENTED_EDGE ( 'NONE', *, *, #9029, .T. ) ;
#11280=ADVANCED_FACE ( 'NONE', ( #4404 ), #6683, .T. ) ;
#11284=ORIENTED_EDGE ( 'NONE', *, *, #2047, .T. ) ;
#11286=ORIENTED_EDGE ( 'NONE', *, *, #14626, .F. ) ;
#11288=PLANE ( 'NONE',  #7366 ) ;
#11289=ORIENTED_EDGE ( 'NONE', *, *, #14306, .F. ) ;
#11290=LINE ( 'NONE', #4102, #11715 ) ;
#11305=VERTEX_POINT ( 'NONE', #922 ) ;
#11306=ORIENTED_EDGE ( 'NONE', *, *, #1445, .F. ) ;
#11317=VECTOR ( 'NONE', #9798, 1000.000000000000000 ) ;
#11321=ORIENTED_EDGE ( 'NONE', *, *, #9725, .T. ) ;
#11325=DIRECTION ( 'NONE',  ( 0.000000000000000000, -1.156482317317871725E-16, 1.000000000000000000 ) ) ;
#11326=ORIENTED_EDGE ( 'NONE', *, *, #2880, .F. ) ;
#11335=AXIS2_PLACEMENT_3D ( 'NONE', #4787, #9612, #5817 ) ;
#11337=CIRCLE ( 'NONE', #8339, 1.699999999999993072 ) ;
#11339=EDGE_LOOP ( 'NONE', ( #11532, #14958, #1636, #7151 ) ) ;
#11342=CARTESIAN_POINT ( 'NONE',  ( 215.1062858801516882, 25.86394065090268057, 18.00000000000000355 ) ) ;
#11349=DIRECTION ( 'NONE',  ( -0.000000000000000000, 1.000000000000000000, 0.000000000000000000 ) ) ;
#11353=CARTESIAN_POINT ( 'NONE',  ( -35.99999999999995026, 59.53993994372674337, 16.70000000000140261 ) ) ;
#11354=DIRECTION ( 'NONE',  ( 0.000000000000000000, 0.000000000000000000, -1.000000000000000000 ) ) ;
#11357=EDGE_CURVE ( 'NONE', #11465, #8395, #8866, .T. ) ;
#11358=ADVANCED_FACE ( 'NONE', ( #677 ), #7432, .T. ) ;
#11366=CIRCLE ( 'NONE', #10106, 3.525000000000000355 ) ;
#11368=DIRECTION ( 'NONE',  ( 0.000000000000000000, 0.000000000000000000, 1.000000000000000000 ) ) ;
#11373=PLANE ( 'NONE',  #8870 ) ;
#11377=AXIS2_PLACEMENT_3D ( 'NONE', #6386, #11194, #13308 ) ;
#11401=DIRECTION ( 'NONE',  ( 0.000000000000000000, -1.000000000000000000, 0.000000000000000000 ) ) ;
#11406=ORIENTED_EDGE ( 'NONE', *, *, #7991, .T. ) ;
#11411=ORIENTED_EDGE ( 'NONE', *, *, #12547, .T. ) ;
#11416=FACE_OUTER_BOUND ( 'NONE', #14085, .T. ) ;
#11421=CARTESIAN_POINT ( 'NONE',  ( 14.00000000000004086, 64.53993994372673626, 15.00000000000104983 ) ) ;
#11424=ORIENTED_EDGE ( 'NONE', *, *, #5368, .T. ) ;
#11426=CARTESIAN_POINT ( 'NONE',  ( 114.0000000000000568, 62.13993994372673768, 16.70000000000034746 ) ) ;
#11429=ORIENTED_EDGE ( 'NONE', *, *, #8860, .F. ) ;
#11436=CARTESIAN_POINT ( 'NONE',  ( 224.0000000000000853, 56.53993994372675047, 25.00000000000000000 ) ) ;
#11439=CARTESIAN_POINT ( 'NONE',  ( -76.50000000000001421, 17.53993994372674692, -17.50000000000002487 ) ) ;
#11446=ADVANCED_FACE ( 'NONE', ( #6147 ), #999, .F. ) ;
#11462=CIRCLE ( 'NONE', #62, 3.525000000000000355 ) ;
#11465=VERTEX_POINT ( 'NONE', #114 ) ;
#11470=ORIENTED_EDGE ( 'NONE', *, *, #747, .F. ) ;
#11476=DIRECTION ( 'NONE',  ( 1.000000000000000000, 0.000000000000000000, 0.000000000000000000 ) ) ;
#11478=EDGE_CURVE ( 'NONE', #12734, #9960, #10648, .T. ) ;
#11479=FACE_OUTER_BOUND ( 'NONE', #7890, .T. ) ;
#11480=DIRECTION ( 'NONE',  ( 0.000000000000000000, 0.000000000000000000, 1.000000000000000000 ) ) ;
#11488=CARTESIAN_POINT ( 'NONE',  ( -85.99999999999994316, 62.13993994372673768, 11.50000000000174438 ) ) ;
#11492=ORIENTED_EDGE ( 'NONE', *, *, #6610, .T. ) ;
#11495=DIRECTION ( 'NONE',  ( 0.000000000000000000, 0.000000000000000000, 1.000000000000000000 ) ) ;
#11496=VECTOR ( 'NONE', #10938, 1000.000000000000000 ) ;
#11497=DIRECTION ( 'NONE',  ( -0.000000000000000000, 1.000000000000000000, -0.000000000000000000 ) ) ;
#11499=EDGE_CURVE ( 'NONE', #14095, #13329, #14877, .T. ) ;
#11502=CARTESIAN_POINT ( 'NONE',  ( 64.00000000000005684, 64.53993994372673626, 15.00000000000070166 ) ) ;
#11509=DIRECTION ( 'NONE',  ( -0.000000000000000000, 1.000000000000000000, -0.000000000000000000 ) ) ;
#11511=VERTEX_POINT ( 'NONE', #10162 ) ;
#11516=DIRECTION ( 'NONE',  ( 0.000000000000000000, 8.673617379884035472E-17, -1.000000000000000000 ) ) ;
#11517=CIRCLE ( 'NONE', #13516, 3.500000000000001332 ) ;
#11528=DIRECTION ( 'NONE',  ( -0.000000000000000000, 1.000000000000000000, -0.000000000000000000 ) ) ;
#11529=DIRECTION ( 'NONE',  ( -0.000000000000000000, 1.000000000000000000, -0.000000000000000000 ) ) ;
#11531=PLANE ( 'NONE',  #12416 ) ;
#11532=ORIENTED_EDGE ( 'NONE', *, *, #3139, .F. ) ;
#11534=ORIENTED_EDGE ( 'NONE', *, *, #1087, .F. ) ;
#11546=CARTESIAN_POINT ( 'NONE',  ( -76.50000000000004263, 17.53993994372673271, 52.49999999999997868 ) ) ;
#11548=CYLINDRICAL_SURFACE ( 'NONE', #12351, 1.699999999999991518 ) ;
#11549=ADVANCED_FACE ( 'NONE', ( #9933 ), #1628, .F. ) ;
#11550=EDGE_CURVE ( 'NONE', #868, #2171, #6693, .T. ) ;
#11565=EDGE_CURVE ( 'NONE', #11151, #259, #6539, .T. ) ;
#11574=DIRECTION ( 'NONE',  ( -0.000000000000000000, 1.000000000000000000, -0.000000000000000000 ) ) ;
#11576=DIRECTION ( 'NONE',  ( 0.000000000000000000, 1.000000000000000000, 0.000000000000000000 ) ) ;
#11584=EDGE_CURVE ( 'NONE', #12466, #11151, #8907, .T. ) ;
#11587=DIRECTION ( 'NONE',  ( -0.000000000000000000, 1.000000000000000000, 1.156482317317871725E-16 ) ) ;
#11596=DIRECTION ( 'NONE',  ( 0.000000000000000000, 1.156482317317871478E-16, -1.000000000000000000 ) ) ;
#11597=CARTESIAN_POINT ( 'NONE',  ( 224.0000000000000853, 22.53993994372673981, 13.00000000000000178 ) ) ;
#11601=CARTESIAN_POINT ( 'NONE',  ( 64.00000000000005684, 56.53993994372675047, 15.00000000000070166 ) ) ;
#11613=ADVANCED_FACE ( 'NONE', ( #499 ), #5340, .F. ) ;
#11616=CIRCLE ( 'NONE', #4806, 1.699999999999993072 ) ;
#11623=DIRECTION ( 'NONE',  ( -0.000000000000000000, 1.000000000000000000, -0.000000000000000000 ) ) ;
#11634=CARTESIAN_POINT ( 'NONE',  ( 224.0000000000000853, 59.53993994372674337, 10.00000000000000178 ) ) ;
#11641=ORIENTED_EDGE ( 'NONE', *, *, #12557, .T. ) ;
#11642=DIRECTION ( 'NONE',  ( 0.000000000000000000, 0.000000000000000000, 1.000000000000000000 ) ) ;
#11648=ORIENTED_EDGE ( 'NONE', *, *, #15038, .F. ) ;
#11652=CIRCLE ( 'NONE', #10383, 1.700000000000007061 ) ;
#11653=DIRECTION ( 'NONE',  ( -0.000000000000000000, 1.000000000000000000, 1.156482317317871725E-16 ) ) ;
#11656=CIRCLE ( 'NONE', #10646, 1.699999999999993072 ) ;
#11657=DIRECTION ( 'NONE',  ( 0.000000000000000000, 0.000000000000000000, 1.000000000000000000 ) ) ;
#11661=AXIS2_PLACEMENT_3D ( 'NONE', #1928, #2093, #4143 ) ;
#11664=DIRECTION ( 'NONE',  ( 0.000000000000000000, 0.000000000000000000, 1.000000000000000000 ) ) ;
#11665=FACE_OUTER_BOUND ( 'NONE', #5507, .T. ) ;
#11666=ORIENTED_EDGE ( 'NONE', *, *, #15038, .T. ) ;
#11667=CLOSED_SHELL ( 'NONE', ( #1428, #9145, #11549, #12119, #5688, #11613, #14051, #11073, #12741, #14492, #1703, #10904, #13424, #11168, #111, #5849, #6484, #5387, #5326, #1541, #6733, #3246, #10595, #6178, #13637, #10144, #14710, #8289, #3549, #2402, #11874, #15468, #6872, #1579, #3439, #13298, #2232, #262, #11740, #6709, #14433, #2477, #15487, #8828, #14393, #6565, #7947, #9399 ) ) ;
#11668=CARTESIAN_POINT ( 'NONE',  ( -85.99999999999994316, 64.53993994372673626, 18.50000000000175149 ) ) ;
#11671=CARTESIAN_POINT ( 'NONE',  ( 190.5000000000000568, 19.53993994372674692, -17.50000000000002487 ) ) ;
#11676=ADVANCED_FACE ( 'NONE', ( #3287 ), #4915, .T. ) ;
#11678=LINE ( 'NONE', #3144, #576 ) ;
#11685=ORIENTED_EDGE ( 'NONE', *, *, #5573, .T. ) ;
#11688=ORIENTED_EDGE ( 'NONE', *, *, #9331, .T. ) ;
#11709=CIRCLE ( 'NONE', #4901, 1.499999999999994449 ) ;
#11712=AXIS2_PLACEMENT_3D ( 'NONE', #2703, #13265, #7524 ) ;
#11715=VECTOR ( 'NONE', #6414, 1000.000000000000000 ) ;
#11717=DIRECTION ( 'NONE',  ( -0.000000000000000000, 1.000000000000000000, -0.000000000000000000 ) ) ;
#11722=VERTEX_POINT ( 'NONE', #12591 ) ;
#11725=ORIENTED_EDGE ( 'NONE', *, *, #15101, .F. ) ;
#11730=VECTOR ( 'NONE', #7002, 1000.000000000000000 ) ;
#11740=ADVANCED_FACE ( 'NONE', ( #6767 ), #741, .F. ) ;
#11741=CARTESIAN_POINT ( 'NONE',  ( -70.00000000000000000, 17.53993994372673981, -13.99999999999999289 ) ) ;
#11744=VERTEX_POINT ( 'NONE', #6850 ) ;
#11746=CARTESIAN_POINT ( 'NONE',  ( -70.00000000000000000, 17.53993994372673271, 47.49999999999997868 ) ) ;
#11752=AXIS2_PLACEMENT_3D ( 'NONE', #4582, #6967, #3558 ) ;
#11758=LINE ( 'NONE', #10809, #4321 ) ;
#11765=CARTESIAN_POINT ( 'NONE',  ( 164.0000000000000568, 64.51493994372674479, 15.00000000000000355 ) ) ;
#11766=AXIS2_PLACEMENT_3D ( 'NONE', #9715, #1169, #7202 ) ;
#11771=ORIENTED_EDGE ( 'NONE', *, *, #13444, .T. ) ;
#11774=ORIENTED_EDGE ( 'NONE', *, *, #2683, .F. ) ;
#11777=CARTESIAN_POINT ( 'NONE',  ( 114.0000000000000568, 64.53993994372673626, 15.00000000000035172 ) ) ;
#11781=FACE_OUTER_BOUND ( 'NONE', #8489, .T. ) ;
#11786=DIRECTION ( 'NONE',  ( -0.000000000000000000, 1.000000000000000000, 1.156482317317871725E-16 ) ) ;
#11789=SURFACE_STYLE_USAGE ( .BOTH. , #6984 ) ;
#11793=CARTESIAN_POINT ( 'NONE',  ( 64.00000000000005684, 59.53993994372674337, 15.00000000000070166 ) ) ;
#11794=ORIENTED_EDGE ( 'NONE', *, *, #6142, .T. ) ;
#11799=ORIENTED_EDGE ( 'NONE', *, *, #12284, .T. ) ;
#11803=CIRCLE ( 'NONE', #13808, 1.699999999999994849 ) ;
#11807=AXIS2_PLACEMENT_3D ( 'NONE', #13619, #5035, #2508 ) ;
#11812=CARTESIAN_POINT ( 'NONE',  ( 200.1062858801516597, 40.86394065090267702, 10.00000000000000000 ) ) ;
#11815=CYLINDRICAL_SURFACE ( 'NONE', #6561, 1.699999999999994849 ) ;
#11820=DIRECTION ( 'NONE',  ( 1.000000000000000000, 0.000000000000000000, 0.000000000000000000 ) ) ;
#11835=VERTEX_POINT ( 'NONE', #4695 ) ;
#11840=EDGE_CURVE ( 'NONE', #9838, #5937, #14973, .T. ) ;
#11843=CARTESIAN_POINT ( 'NONE',  ( 0.000000000000000000, 0.000000000000000000, 18.00000000000000355 ) ) ;
#11853=CARTESIAN_POINT ( 'NONE',  ( 14.00000000000004086, 56.53993994372675047, 13.30000000000105231 ) ) ;
#11856=FACE_OUTER_BOUND ( 'NONE', #5665, .T. ) ;
#11857=ORIENTED_EDGE ( 'NONE', *, *, #917, .T. ) ;
#11864=AXIS2_PLACEMENT_3D ( 'NONE', #5778, #8010, #14141 ) ;
#11865=AXIS2_PLACEMENT_3D ( 'NONE', #10415, #3309, #8144 ) ;
#11866=CIRCLE ( 'NONE', #12360, 4.999999999999990230 ) ;
#11867=DIRECTION ( 'NONE',  ( 0.000000000000000000, 0.000000000000000000, -1.000000000000000000 ) ) ;
#11869=LINE ( 'NONE', #3343, #993 ) ;
#11874=ADVANCED_FACE ( 'NONE', ( #14316 ), #14398, .F. ) ;
#11882=CARTESIAN_POINT ( 'NONE',  ( 114.0000000000000568, 64.53993994372673626, 16.70000000000034746 ) ) ;
#11885=VECTOR ( 'NONE', #792, 1000.000000000000000 ) ;
#11892=DIRECTION ( 'NONE',  ( -0.000000000000000000, 1.000000000000000000, -0.000000000000000000 ) ) ;
#11893=DIRECTION ( 'NONE',  ( -0.000000000000000000, 1.000000000000000000, -0.000000000000000000 ) ) ;
#11894=VECTOR ( 'NONE', #5290, 1000.000000000000000 ) ;
#11895=FACE_BOUND ( 'NONE', #3727, .T. ) ;
#11909=DIRECTION ( 'NONE',  ( -0.000000000000000000, 1.000000000000000000, -0.000000000000000000 ) ) ;
#11910=CARTESIAN_POINT ( 'NONE',  ( -70.00000000000000000, 17.53993994372673271, 47.49999999999997868 ) ) ;
#11918=FACE_OUTER_BOUND ( 'NONE', #12675, .T. ) ;
#11923=VERTEX_POINT ( 'NONE', #10785 ) ;
#11929=ORIENTED_EDGE ( 'NONE', *, *, #7863, .T. ) ;
#11934=EDGE_CURVE ( 'NONE', #1467, #11722, #1065, .T. ) ;
#11935=VERTEX_POINT ( 'NONE', #15420 ) ;
#11937=CARTESIAN_POINT ( 'NONE',  ( 177.5000000000000853, 19.53993994372674692, -17.50000000000002487 ) ) ;
#11938=EDGE_LOOP ( 'NONE', ( #13233, #12785, #4946, #3407 ) ) ;
#11940=DIRECTION ( 'NONE',  ( 0.000000000000000000, -1.000000000000000000, 0.000000000000000000 ) ) ;
#11942=CONICAL_SURFACE ( 'NONE', #5133, 3.525000000000000355, 0.7853981633975176679 ) ;
#11946=PLANE ( 'NONE',  #4015 ) ;
#11949=VERTEX_POINT ( 'NONE', #4619 ) ;
#11959=LINE ( 'NONE', #11882, #5031 ) ;
#11963=EDGE_LOOP ( 'NONE', ( #8297, #1817, #6401, #12324 ) ) ;
#11970=DIRECTION ( 'NONE',  ( 0.000000000000000000, 0.000000000000000000, 1.000000000000000000 ) ) ;
#11972=FACE_OUTER_BOUND ( 'NONE', #210, .T. ) ;
#11985=ADVANCED_FACE ( 'NONE', ( #11097 ), #252, .F. ) ;
#11987=DIRECTION ( 'NONE',  ( -0.000000000000000000, 1.000000000000000000, -0.000000000000000000 ) ) ;
#11988=DIRECTION ( 'NONE',  ( 0.000000000000000000, -0.000000000000000000, 1.000000000000000000 ) ) ;
#11991=CARTESIAN_POINT ( 'NONE',  ( -110.0000000000000426, 56.53993994372675047, 13.00000000000000178 ) ) ;
#11992=ORIENTED_EDGE ( 'NONE', *, *, #7642, .F. ) ;
#11995=DIRECTION ( 'NONE',  ( 0.000000000000000000, -1.000000000000000000, 0.000000000000000000 ) ) ;
#11997=SURFACE_SIDE_STYLE ('',( #6083 ) ) ;
#12003=AXIS2_PLACEMENT_3D ( 'NONE', #7308, #8495, #13277 ) ;
#12004=ORIENTED_EDGE ( 'NONE', *, *, #3532, .F. ) ;
#12017=DIRECTION ( 'NONE',  ( 3.965082230804130220E-16, 1.486905836551548832E-16, -1.000000000000000000 ) ) ;
#12021=CARTESIAN_POINT ( 'NONE',  ( 64.00000000000005684, 56.53993994372675047, 13.30000000000070948 ) ) ;
#12023=ORIENTED_EDGE ( 'NONE', *, *, #7417, .T. ) ;
#12024=VERTEX_POINT ( 'NONE', #3834 ) ;
#12031=FACE_OUTER_BOUND ( 'NONE', #15535, .T. ) ;
#12034=ORIENTED_EDGE ( 'NONE', *, *, #1251, .T. ) ;
#12045=ORIENTED_EDGE ( 'NONE', *, *, #9245, .T. ) ;
#12054=FACE_OUTER_BOUND ( 'NONE', #382, .T. ) ;
#12066=CARTESIAN_POINT ( 'NONE',  ( 184.0000000000000568, 19.53993994372673626, 48.99999999999997158 ) ) ;
#12068=CYLINDRICAL_SURFACE ( 'NONE', #3120, 1.499999999999997780 ) ;
#12080=EDGE_LOOP ( 'NONE', ( #13155, #10171, #11289, #4328 ) ) ;
#12091=EDGE_CURVE ( 'NONE', #12821, #2912, #6189, .T. ) ;
#12092=VERTEX_POINT ( 'NONE', #646 ) ;
#12098=CIRCLE ( 'NONE', #5294, 1.700000000000000178 ) ;
#12099=VERTEX_POINT ( 'NONE', #2075 ) ;
#12107=AXIS2_PLACEMENT_3D ( 'NONE', #7136, #11940, #5932 ) ;
#12118=EDGE_CURVE ( 'NONE', #5947, #10243, #8222, .T. ) ;
#12119=ADVANCED_FACE ( 'NONE', ( #6907 ), #1377, .F. ) ;
#12122=DIRECTION ( 'NONE',  ( -0.000000000000000000, 1.000000000000000000, -0.000000000000000000 ) ) ;
#12129=VECTOR ( 'NONE', #5308, 1000.000000000000000 ) ;
#12136=EDGE_CURVE ( 'NONE', #11949, #15030, #15017, .T. ) ;
#12142=LINE ( 'NONE', #6080, #10285 ) ;
#12147=DIRECTION ( 'NONE',  ( 0.000000000000000000, -1.000000000000000000, 0.000000000000000000 ) ) ;
#12148=DIRECTION ( 'NONE',  ( -0.000000000000000000, 1.000000000000000000, -0.000000000000000000 ) ) ;
#12154=CYLINDRICAL_SURFACE ( 'NONE', #15156, 1.499999999999994449 ) ;
#12155=EDGE_LOOP ( 'NONE', ( #7734, #15612 ) ) ;
#12156=VECTOR ( 'NONE', #402, 1000.000000000000000 ) ;
#12160=AXIS2_PLACEMENT_3D ( 'NONE', #10345, #9171, #13971 ) ;
#12162=ORIENTED_EDGE ( 'NONE', *, *, #11075, .T. ) ;
#12165=CYLINDRICAL_SURFACE ( 'NONE', #1069, 3.500000000000003109 ) ;
#12195=VECTOR ( 'NONE', #14485, 1000.000000000000000 ) ;
#12198=DIRECTION ( 'NONE',  ( 3.965082230804130220E-16, -1.486905836551548832E-16, 1.000000000000000000 ) ) ;
#12210=DIRECTION ( 'NONE',  ( -0.000000000000000000, 1.000000000000000000, -0.000000000000000000 ) ) ;
#12221=FACE_OUTER_BOUND ( 'NONE', #13331, .T. ) ;
#12224=EDGE_CURVE ( 'NONE', #14758, #7532, #3649, .T. ) ;
#12230=ORIENTED_EDGE ( 'NONE', *, *, #12557, .F. ) ;
#12232=ORIENTED_EDGE ( 'NONE', *, *, #4164, .F. ) ;
#12240=CARTESIAN_POINT ( 'NONE',  ( 114.0000000000000568, 56.53993994372675047, 16.70000000000034746 ) ) ;
#12245=LINE ( 'NONE', #8780, #14355 ) ;
#12255=FACE_OUTER_BOUND ( 'NONE', #1391, .T. ) ;
#12256=DIRECTION ( 'NONE',  ( 1.000000000000000000, 0.000000000000000000, 0.000000000000000000 ) ) ;
#12257=DIRECTION ( 'NONE',  ( -0.000000000000000000, 1.000000000000000000, -0.000000000000000000 ) ) ;
#12258=VECTOR ( 'NONE', #10718, 1000.000000000000000 ) ;
#12259=FACE_BOUND ( 'NONE', #9883, .T. ) ;
#12263=CARTESIAN_POINT ( 'NONE',  ( 185.1062858801516882, 55.86394065090267702, 18.00000000000000355 ) ) ;
#12266=LINE ( 'NONE', #6284, #9555 ) ;
#12267=ORIENTED_EDGE ( 'NONE', *, *, #8427, .T. ) ;
#12277=CARTESIAN_POINT ( 'NONE',  ( 215.1062858801516882, 25.86394065090268057, 18.00000000000000355 ) ) ;
#12280=CARTESIAN_POINT ( 'NONE',  ( 200.1062858801516597, 40.86394065090267702, 10.00000000000000000 ) ) ;
#12284=EDGE_CURVE ( 'NONE', #5947, #12618, #14150, .T. ) ;
#12292=CARTESIAN_POINT ( 'NONE',  ( -70.00000000000000000, 17.53993994372673981, -12.49999999999999467 ) ) ;
#12297=VECTOR ( 'NONE', #5594, 1000.000000000000000 ) ;
#12298=CARTESIAN_POINT ( 'NONE',  ( 114.0000000000000568, 59.53993994372674337, 16.70000000000034746 ) ) ;
#12299=CONICAL_SURFACE ( 'NONE', #12802, 3.525000000000002132, 0.7853981633974482790 ) ;
#12300=VECTOR ( 'NONE', #14494, 1000.000000000000000 ) ;
#12301=CARTESIAN_POINT ( 'NONE',  ( -85.99999999999994316, 64.53993994372673626, 13.30000000000175575 ) ) ;
#12324=ORIENTED_EDGE ( 'NONE', *, *, #14236, .T. ) ;
#12337=AXIS2_PLACEMENT_3D ( 'NONE', #4568, #8147, #5681 ) ;
#12343=FACE_BOUND ( 'NONE', #9166, .T. ) ;
#12345=COLOUR_RGB ( '', 0.72549020, 0.75294118, 0.79215686) ;
#12351=AXIS2_PLACEMENT_3D ( 'NONE', #6748, #3414, #12799 ) ;
#12354=ORIENTED_EDGE ( 'NONE', *, *, #2804, .T. ) ;
#12355=DIRECTION ( 'NONE',  ( 0.000000000000000000, 0.000000000000000000, 1.000000000000000000 ) ) ;
#12357=VECTOR ( 'NONE', #5863, 1000.000000000000000 ) ;
#12359=VECTOR ( 'NONE', #1939, 1000.000000000000000 ) ;
#12360=AXIS2_PLACEMENT_3D ( 'NONE', #8981, #13774, #8817 ) ;
#12363=DIRECTION ( 'NONE',  ( -0.000000000000000000, 1.000000000000000000, -0.000000000000000000 ) ) ;
#12364=DIRECTION ( 'NONE',  ( -0.000000000000000000, -8.673617379884035472E-17, 1.000000000000000000 ) ) ;
#12366=DIRECTION ( 'NONE',  ( -0.000000000000000000, 1.000000000000000000, 1.156482317317871725E-16 ) ) ;
#12368=DIRECTION ( 'NONE',  ( -0.000000000000000000, 1.000000000000000000, 0.000000000000000000 ) ) ;
#12370=ORIENTED_EDGE ( 'NONE', *, *, #11499, .T. ) ;
#12375=DIRECTION ( 'NONE',  ( -0.000000000000000000, -1.000000000000000000, -0.000000000000000000 ) ) ;
#12380=CIRCLE ( 'NONE', #4828, 1.700000000000000178 ) ;
#12394=CARTESIAN_POINT ( 'NONE',  ( -76.50000000000004263, 19.53993994372673626, 52.49999999999997868 ) ) ;
#12397=ORIENTED_EDGE ( 'NONE', *, *, #5615, .F. ) ;
#12399=EDGE_CURVE ( 'NONE', #12092, #13079, #10739, .T. ) ;
#12401=EDGE_LOOP ( 'NONE', ( #10981, #6406, #10610, #3100 ) ) ;
#12402=CARTESIAN_POINT ( 'NONE',  ( 14.00000000000004086, 62.13993994372673768, 15.00000000000104983 ) ) ;
#12404=DIRECTION ( 'NONE',  ( -0.000000000000000000, 1.000000000000000000, 1.156482317317871725E-16 ) ) ;
#12409=ORIENTED_EDGE ( 'NONE', *, *, #3050, .F. ) ;
#12416=AXIS2_PLACEMENT_3D ( 'NONE', #9014, #15222, #12859 ) ;
#12420=ORIENTED_EDGE ( 'NONE', *, *, #2507, .F. ) ;
#12427=CIRCLE ( 'NONE', #2611, 1.699999999999998401 ) ;
#12429=EDGE_CURVE ( 'NONE', #9960, #627, #4422, .T. ) ;
#12434=CIRCLE ( 'NONE', #10695, 1.499999999999994449 ) ;
#12436=ORIENTED_EDGE ( 'NONE', *, *, #2176, .F. ) ;
#12438=CONICAL_SURFACE ( 'NONE', #2113, 3.525000000000000355, 0.7853981633974482790 ) ;
#12440=DIRECTION ( 'NONE',  ( -0.000000000000000000, 1.000000000000000000, -0.000000000000000000 ) ) ;
#12443=CARTESIAN_POINT ( 'NONE',  ( 190.5000000000000853, 17.53993994372673271, 52.49999999999997868 ) ) ;
#12444=AXIS2_PLACEMENT_3D ( 'NONE', #4466, #3067, #668 ) ;
#12450=CONICAL_SURFACE ( 'NONE', #10947, 3.525000000000002132, 0.7853981633974482790 ) ;
#12452=( LENGTH_UNIT ( ) NAMED_UNIT ( * ) SI_UNIT ( .MILLI., .METRE. ) );
#12457=ORIENTED_EDGE ( 'NONE', *, *, #11934, .F. ) ;
#12466=VERTEX_POINT ( 'NONE', #2867 ) ;
#12470=CARTESIAN_POINT ( 'NONE',  ( -76.50000000000001421, 19.53993994372674692, -17.50000000000002487 ) ) ;
#12473=ORIENTED_EDGE ( 'NONE', *, *, #5362, .F. ) ;
#12475=CARTESIAN_POINT ( 'NONE',  ( 14.00000000000004086, 59.53993994372674337, 16.70000000000104734 ) ) ;
#12479=CARTESIAN_POINT ( 'NONE',  ( 14.00000000000004086, 62.13993994372673768, 18.50000000000105160 ) ) ;
#12487=CYLINDRICAL_SURFACE ( 'NONE', #2273, 3.499999999999999556 ) ;
#12490=DIRECTION ( 'NONE',  ( 1.000000000000000000, 0.000000000000000000, 0.000000000000000000 ) ) ;
#12491=AXIS2_PLACEMENT_3D ( 'NONE', #1668, #8000, #12709 ) ;
#12493=CARTESIAN_POINT ( 'NONE',  ( -110.0000000000000426, 56.53993994372675047, 25.00000000000000000 ) ) ;
#12506=CIRCLE ( 'NONE', #3181, 3.500000000000003109 ) ;
#12511=VECTOR ( 'NONE', #9475, 1000.000000000000000 ) ;
#12519=ORIENTED_EDGE ( 'NONE', *, *, #5368, .F. ) ;
#12527=ADVANCED_FACE ( 'NONE', ( #7689 ), #5469, .F. ) ;
#12531=CARTESIAN_POINT ( 'NONE',  ( 215.1062858801516882, 25.86394065090268057, 13.00000000000000178 ) ) ;
#12539=CARTESIAN_POINT ( 'NONE',  ( -108.0000000000000568, 59.53993994372674337, 10.00000000000000178 ) ) ;
#12547=EDGE_CURVE ( 'NONE', #8130, #319, #9230, .T. ) ;
#12548=PRODUCT_CONTEXT ( 'NONE', #5649, 'mechanical' ) ;
#12551=ORIENTED_EDGE ( 'NONE', *, *, #9134, .F. ) ;
#12553=CARTESIAN_POINT ( 'NONE',  ( -35.99999999999995026, 64.53993994372673626, 15.00000000000139977 ) ) ;
#12554=ORIENTED_EDGE ( 'NONE', *, *, #5274, .F. ) ;
#12555=ORIENTED_EDGE ( 'NONE', *, *, #855, .F. ) ;
#12557=EDGE_CURVE ( 'NONE', #6601, #10382, #6664, .T. ) ;
#12560=CARTESIAN_POINT ( 'NONE',  ( 177.5000000000000853, 17.53993994372674692, -17.50000000000002487 ) ) ;
#12564=CARTESIAN_POINT ( 'NONE',  ( 64.00000000000005684, 59.53993994372674337, 16.70000000000069207 ) ) ;
#12567=DIRECTION ( 'NONE',  ( 0.000000000000000000, 0.000000000000000000, -1.000000000000000000 ) ) ;
#12568=ORIENTED_EDGE ( 'NONE', *, *, #2084, .T. ) ;
#12591=CARTESIAN_POINT ( 'NONE',  ( 224.0000000000000853, 19.53993994372674337, 9.999999999999998224 ) ) ;
#12598=ORIENTED_EDGE ( 'NONE', *, *, #11478, .T. ) ;
#12603=AXIS2_PLACEMENT_3D ( 'NONE', #608, #15281, #2117 ) ;
#12614=CARTESIAN_POINT ( 'NONE',  ( 164.0000000000000568, 64.53993994372673626, 15.00000000000000355 ) ) ;
#12615=VECTOR ( 'NONE', #14884, 1000.000000000000000 ) ;
#12618=VERTEX_POINT ( 'NONE', #5301 ) ;
#12622=DIRECTION ( 'NONE',  ( -0.000000000000000000, 1.000000000000000000, 0.000000000000000000 ) ) ;
#12623=CARTESIAN_POINT ( 'NONE',  ( -63.50000000000002842, 19.53993994372674337, 24.99999999999999645 ) ) ;
#12626=CARTESIAN_POINT ( 'NONE',  ( -70.00000000000000000, 19.53993994372673626, 45.99999999999998579 ) ) ;
#12627=AXIS2_PLACEMENT_3D ( 'NONE', #5812, #9686, #14320 ) ;
#12632=ORIENTED_EDGE ( 'NONE', *, *, #11584, .F. ) ;
#12634=LINE ( 'NONE', #308, #936 ) ;
#12637=AXIS2_PLACEMENT_3D ( 'NONE', #1322, #6231, #8524 ) ;
#12638=CARTESIAN_POINT ( 'NONE',  ( 64.00000000000005684, 59.53993994372674337, 13.30000000000070948 ) ) ;
#12642=FACE_OUTER_BOUND ( 'NONE', #1743, .T. ) ;
#12645=PLANE ( 'NONE',  #10079 ) ;
#12650=DIRECTION ( 'NONE',  ( 0.000000000000000000, 0.000000000000000000, 1.000000000000000000 ) ) ;
#12662=LINE ( 'NONE', #2004, #14592 ) ;
#12664=DIRECTION ( 'NONE',  ( 1.000000000000000000, 0.000000000000000000, 0.000000000000000000 ) ) ;
#12669=CYLINDRICAL_SURFACE ( 'NONE', #13044, 1.700000000000007061 ) ;
#12674=DIRECTION ( 'NONE',  ( -0.000000000000000000, 1.000000000000000000, -0.000000000000000000 ) ) ;
#12675=EDGE_LOOP ( 'NONE', ( #1209, #12023 ) ) ;
#12691=EDGE_LOOP ( 'NONE', ( #1023, #14044, #10913, #2750, #2382, #8829 ) ) ;
#12693=VERTEX_POINT ( 'NONE', #941 ) ;
#12695=FACE_BOUND ( 'NONE', #2158, .T. ) ;
#12696=EDGE_CURVE ( 'NONE', #14095, #2217, #10990, .T. ) ;
#12699=ADVANCED_FACE ( 'NONE', ( #2134 ), #865, .F. ) ;
#12702=FACE_BOUND ( 'NONE', #7039, .T. ) ;
#12703=EDGE_LOOP ( 'NONE', ( #2127, #12632, #2133, #8128 ) ) ;
#12709=DIRECTION ( 'NONE',  ( 0.000000000000000000, 0.000000000000000000, -1.000000000000000000 ) ) ;
#12716=ORIENTED_EDGE ( 'NONE', *, *, #11565, .T. ) ;
#12718=CARTESIAN_POINT ( 'NONE',  ( 164.0000000000000568, 64.53993994372673626, 16.70000000000000995 ) ) ;
#12719=CARTESIAN_POINT ( 'NONE',  ( -70.00000000000000000, 19.53993994372673626, 47.49999999999997868 ) ) ;
#12720=CARTESIAN_POINT ( 'NONE',  ( -110.0000000000000426, 19.53993994372674337, 24.99999999999999645 ) ) ;
#12729=LINE ( 'NONE', #4286, #9311 ) ;
#12734=VERTEX_POINT ( 'NONE', #7045 ) ;
#12741=ADVANCED_FACE ( 'NONE', ( #14205 ), #3403, .F. ) ;
#12743=CARTESIAN_POINT ( 'NONE',  ( 14.00000000000004086, 64.51493994372674479, 15.00000000000104983 ) ) ;
#12744=EDGE_CURVE ( 'NONE', #973, #9587, #12868, .T. ) ;
#12753=ORIENTED_EDGE ( 'NONE', *, *, #8531, .F. ) ;
#12758=CARTESIAN_POINT ( 'NONE',  ( 164.0000000000000568, 62.13993994372673768, 16.70000000000000995 ) ) ;
#12761=DIRECTION ( 'NONE',  ( 0.000000000000000000, 0.000000000000000000, 1.000000000000000000 ) ) ;
#12762=AXIS2_PLACEMENT_3D ( 'NONE', #9173, #7990, #12776 ) ;
#12766=EDGE_CURVE ( 'NONE', #3817, #10635, #7475, .T. ) ;
#12772=DIRECTION ( 'NONE',  ( 0.000000000000000000, 0.000000000000000000, 1.000000000000000000 ) ) ;
#12776=DIRECTION ( 'NONE',  ( 0.000000000000000000, -0.000000000000000000, -1.000000000000000000 ) ) ;
#12778=EDGE_LOOP ( 'NONE', ( #4980, #3998, #504, #11857 ) ) ;
#12779=VERTEX_POINT ( 'NONE', #11436 ) ;
#12785=ORIENTED_EDGE ( 'NONE', *, *, #13444, .F. ) ;
#12791=DIRECTION ( 'NONE',  ( 0.000000000000000000, 0.000000000000000000, -1.000000000000000000 ) ) ;
#12799=DIRECTION ( 'NONE',  ( 0.000000000000000000, 0.000000000000000000, 1.000000000000000000 ) ) ;
#12801=FACE_BOUND ( 'NONE', #4548, .T. ) ;
#12802=AXIS2_PLACEMENT_3D ( 'NONE', #12553, #5546, #786 ) ;
#12816=AXIS2_PLACEMENT_3D ( 'NONE', #15271, #7009, #14021 ) ;
#12821=VERTEX_POINT ( 'NONE', #5357 ) ;
#12830=CARTESIAN_POINT ( 'NONE',  ( -35.99999999999995026, 62.13993994372673768, 15.00000000000139977 ) ) ;
#12844=LINE ( 'NONE', #15127, #13687 ) ;
#12848=DIRECTION ( 'NONE',  ( -0.000000000000000000, 1.000000000000000000, 0.000000000000000000 ) ) ;
#12859=DIRECTION ( 'NONE',  ( 0.000000000000000000, 1.486905836551548832E-16, -1.000000000000000000 ) ) ;
#12862=AXIS2_PLACEMENT_3D ( 'NONE', #7797, #11497, #4067 ) ;
#12868=LINE ( 'NONE', #3475, #6213 ) ;
#12869=DIRECTION ( 'NONE',  ( 0.000000000000000000, -1.000000000000000000, -1.156482317317871478E-16 ) ) ;
#12871=VECTOR ( 'NONE', #13806, 1000.000000000000000 ) ;
#12872=ORIENTED_EDGE ( 'NONE', *, *, #1908, .F. ) ;
#12876=DIRECTION ( 'NONE',  ( 0.000000000000000000, 1.486905836551548832E-16, -1.000000000000000000 ) ) ;
#12883=DIRECTION ( 'NONE',  ( 0.000000000000000000, 0.000000000000000000, 1.000000000000000000 ) ) ;
#12886=CYLINDRICAL_SURFACE ( 'NONE', #6311, 3.500000000000001332 ) ;
#12889=DIRECTION ( 'NONE',  ( -0.000000000000000000, 1.000000000000000000, -0.000000000000000000 ) ) ;
#12898=DIRECTION ( 'NONE',  ( 0.000000000000000000, 1.156482317317871725E-16, -1.000000000000000000 ) ) ;
#12902=AXIS2_PLACEMENT_3D ( 'NONE', #11601, #14975, #9083 ) ;
#12903=DIRECTION ( 'NONE',  ( -0.000000000000000000, 1.000000000000000000, -0.000000000000000000 ) ) ;
#12906=DIRECTION ( 'NONE',  ( 1.000000000000000000, 0.000000000000000000, 0.000000000000000000 ) ) ;
#12907=ORIENTED_EDGE ( 'NONE', *, *, #3722, .F. ) ;
#12910=FACE_BOUND ( 'NONE', #14612, .T. ) ;
#12912=ORIENTED_EDGE ( 'NONE', *, *, #4815, .T. ) ;
#12915=EDGE_CURVE ( 'NONE', #3955, #4984, #10177, .T. ) ;
#12920=CARTESIAN_POINT ( 'NONE',  ( 114.0000000000000568, 64.53993994372673626, 15.00000000000035172 ) ) ;
#12929=LINE ( 'NONE', #11991, #15413 ) ;
#12933=CARTESIAN_POINT ( 'NONE',  ( -85.99999999999994316, 64.51493994372674479, 11.50000000000174438 ) ) ;
#12936=DIRECTION ( 'NONE',  ( -0.000000000000000000, 1.000000000000000000, -0.000000000000000000 ) ) ;
#12938=AXIS2_PLACEMENT_3D ( 'NONE', #755, #4314, #6941 ) ;
#12945=DIRECTION ( 'NONE',  ( 0.000000000000000000, -1.000000000000000000, 0.000000000000000000 ) ) ;
#12947=DIRECTION ( 'NONE',  ( 0.000000000000000000, 0.000000000000000000, -1.000000000000000000 ) ) ;
#12950=ORIENTED_EDGE ( 'NONE', *, *, #13462, .T. ) ;
#12951=CARTESIAN_POINT ( 'NONE',  ( -35.99999999999995026, 59.53993994372674337, 15.00000000000139977 ) ) ;
#12952=DIRECTION ( 'NONE',  ( -0.000000000000000000, 1.000000000000000000, -0.000000000000000000 ) ) ;
#12953=ORIENTED_EDGE ( 'NONE', *, *, #4835, .F. ) ;
#12959=AXIS2_PLACEMENT_3D ( 'NONE', #12539, #1732, #10037 ) ;
#12961=ORIENTED_EDGE ( 'NONE', *, *, #244, .F. ) ;
#12963=VECTOR ( 'NONE', #4638, 1000.000000000000000 ) ;
#12973=CARTESIAN_POINT ( 'NONE',  ( 215.1062858801516882, 55.86394065090267702, 18.00000000000000355 ) ) ;
#12980=VERTEX_POINT ( 'NONE', #3071 ) ;
#12999=DIRECTION ( 'NONE',  ( 3.965082230804130220E-16, 1.486905836551548832E-16, -1.000000000000000000 ) ) ;
#13000=CARTESIAN_POINT ( 'NONE',  ( 64.00000000000005684, 62.13993994372673768, 15.00000000000070166 ) ) ;
#13008=DIRECTION ( 'NONE',  ( 0.000000000000000000, 0.000000000000000000, 1.000000000000000000 ) ) ;
#13017=CARTESIAN_POINT ( 'NONE',  ( 177.5000000000000853, 19.53993994372674337, 9.999999999999998224 ) ) ;
#13038=CARTESIAN_POINT ( 'NONE',  ( 224.0000000000000853, 56.53993994372675047, 25.00000000000000000 ) ) ;
#13044=AXIS2_PLACEMENT_3D ( 'NONE', #15112, #10318, #2977 ) ;
#13055=VERTEX_POINT ( 'NONE', #7019 ) ;
#13068=LINE ( 'NONE', #3684, #5901 ) ;
#13069=AXIS2_PLACEMENT_3D ( 'NONE', #613, #12622, #12772 ) ;
#13070=ADVANCED_FACE ( 'NONE', ( #363 ), #5049, .F. ) ;
#13079=VERTEX_POINT ( 'NONE', #12298 ) ;
#13086=EDGE_CURVE ( 'NONE', #4984, #10665, #7745, .T. ) ;
#13109=LINE ( 'NONE', #2385, #15176 ) ;
#13117=EDGE_CURVE ( 'NONE', #5937, #12099, #14193, .T. ) ;
#13118=LINE ( 'NONE', #14152, #5026 ) ;
#13119=ORIENTED_EDGE ( 'NONE', *, *, #1880, .T. ) ;
#13126=AXIS2_PLACEMENT_3D ( 'NONE', #9110, #8090, #12876 ) ;
#13139=DIRECTION ( 'NONE',  ( -0.000000000000000000, -1.000000000000000000, -0.000000000000000000 ) ) ;
#13143=FACE_BOUND ( 'NONE', #10167, .T. ) ;
#13154=CARTESIAN_POINT ( 'NONE',  ( -110.0000000000000426, 56.53993994372675047, 13.00000000000000178 ) ) ;
#13155=ORIENTED_EDGE ( 'NONE', *, *, #8002, .T. ) ;
#13162=DIRECTION ( 'NONE',  ( -0.000000000000000000, 1.000000000000000000, -0.000000000000000000 ) ) ;
#13164=CIRCLE ( 'NONE', #7644, 1.699999999999998401 ) ;
#13168=EDGE_LOOP ( 'NONE', ( #4819, #12420, #4424, #14656 ) ) ;
#13174=EDGE_CURVE ( 'NONE', #8543, #4053, #12844, .T. ) ;
#13175=ADVANCED_FACE ( 'NONE', ( #9231 ), #2031, .T. ) ;
#13196=ORIENTED_EDGE ( 'NONE', *, *, #14332, .T. ) ;
#13197=AXIS2_PLACEMENT_3D ( 'NONE', #2204, #15372, #5915 ) ;
#13201=EDGE_CURVE ( 'NONE', #4775, #7275, #2359, .T. ) ;
#13206=CIRCLE ( 'NONE', #13711, 1.700000000000000178 ) ;
#13209=ORIENTED_EDGE ( 'NONE', *, *, #9420, .F. ) ;
#13225=EDGE_CURVE ( 'NONE', #9422, #6607, #11678, .T. ) ;
#13227=DIRECTION ( 'NONE',  ( -0.000000000000000000, 1.000000000000000000, -0.000000000000000000 ) ) ;
#13231=CARTESIAN_POINT ( 'NONE',  ( -35.99999999999995026, 56.53993994372675047, 16.70000000000140261 ) ) ;
#13233=ORIENTED_EDGE ( 'NONE', *, *, #3272, .T. ) ;
#13234=EDGE_CURVE ( 'NONE', #10742, #12734, #12427, .T. ) ;
#13236=ORIENTED_EDGE ( 'NONE', *, *, #2371, .T. ) ;
#13259=DIRECTION ( 'NONE',  ( 0.000000000000000000, 0.000000000000000000, 1.000000000000000000 ) ) ;
#13265=DIRECTION ( 'NONE',  ( 0.000000000000000000, -1.000000000000000000, -1.156482317317871478E-16 ) ) ;
#13266=EDGE_CURVE ( 'NONE', #12618, #9525, #4370, .T. ) ;
#13268=DIRECTION ( 'NONE',  ( -0.000000000000000000, 1.000000000000000000, -0.000000000000000000 ) ) ;
#13275=ORIENTED_EDGE ( 'NONE', *, *, #253, .T. ) ;
#13277=DIRECTION ( 'NONE',  ( 0.000000000000000000, -0.000000000000000000, 1.000000000000000000 ) ) ;
#13279=ADVANCED_FACE ( 'NONE', ( #10889 ), #3612, .F. ) ;
#13283=ORIENTED_EDGE ( 'NONE', *, *, #6341, .T. ) ;
#13287=ADVANCED_FACE ( 'NONE', ( #14181 ), #5982, .T. ) ;
#13294=ORIENTED_EDGE ( 'NONE', *, *, #2642, .T. ) ;
#13297=CARTESIAN_POINT ( 'NONE',  ( -35.99999999999995026, 64.53993994372673626, 11.47500000000139941 ) ) ;
#13298=ADVANCED_FACE ( 'NONE', ( #12054 ), #11942, .F. ) ;
#13301=CARTESIAN_POINT ( 'NONE',  ( 200.1062858801516597, 40.86394065090267702, 16.00000000000001421 ) ) ;
#13304=DIRECTION ( 'NONE',  ( 1.000000000000000000, 0.000000000000000000, 0.000000000000000000 ) ) ;
#13308=DIRECTION ( 'NONE',  ( 0.000000000000000000, 0.000000000000000000, 1.000000000000000000 ) ) ;
#13310=VERTEX_POINT ( 'NONE', #7259 ) ;
#13312=VECTOR ( 'NONE', #13537, 1000.000000000000000 ) ;
#13316=CARTESIAN_POINT ( 'NONE',  ( 114.0000000000000568, 62.13993994372673768, 13.30000000000035776 ) ) ;
#13318=CARTESIAN_POINT ( 'NONE',  ( 184.0000000000000568, 17.53993994372673981, -12.49999999999999467 ) ) ;
#13321=LINE ( 'NONE', #14504, #8079 ) ;
#13325=AXIS2_PLACEMENT_3D ( 'NONE', #15500, #3441, #9291 ) ;
#13329=VERTEX_POINT ( 'NONE', #4713 ) ;
#13331=EDGE_LOOP ( 'NONE', ( #8800, #66, #11253, #6809 ) ) ;
#13334=AXIS2_PLACEMENT_3D ( 'NONE', #10779, #14541, #5007 ) ;
#13335=CIRCLE ( 'NONE', #6290, 1.700000000000007061 ) ;
#13337=ORIENTED_EDGE ( 'NONE', *, *, #856, .F. ) ;
#13340=FACE_OUTER_BOUND ( 'NONE', #9668, .T. ) ;
#13341=ORIENTED_EDGE ( 'NONE', *, *, #6901, .F. ) ;
#13343=AXIS2_PLACEMENT_3D ( 'NONE', #1248, #12148, #1326 ) ;
#13345=ORIENTED_EDGE ( 'NONE', *, *, #4302, .F. ) ;
#13349=CARTESIAN_POINT ( 'NONE',  ( 114.0000000000000568, 59.53993994372674337, 15.00000000000035172 ) ) ;
#13356=CIRCLE ( 'NONE', #12603, 4.999999999999990230 ) ;
#13360=EDGE_CURVE ( 'NONE', #5662, #13310, #3630, .T. ) ;
#13366=VECTOR ( 'NONE', #6029, 1000.000000000000000 ) ;
#13370=LINE ( 'NONE', #8502, #14148 ) ;
#13374=ORIENTED_EDGE ( 'NONE', *, *, #2683, .T. ) ;
#13377=EDGE_CURVE ( 'NONE', #8299, #5720, #13068, .T. ) ;
#13379=ORIENTED_EDGE ( 'NONE', *, *, #8462, .F. ) ;
#13384=AXIS2_PLACEMENT_3D ( 'NONE', #10283, #4268, #12791 ) ;
#13394=CYLINDRICAL_SURFACE ( 'NONE', #10119, 1.499999999999997780 ) ;
#13396=DIRECTION ( 'NONE',  ( -0.000000000000000000, 1.000000000000000000, -0.000000000000000000 ) ) ;
#13403=VECTOR ( 'NONE', #1647, 1000.000000000000000 ) ;
#13404=FACE_OUTER_BOUND ( 'NONE', #86, .T. ) ;
#13408=CARTESIAN_POINT ( 'NONE',  ( 177.5000000000000853, 17.53993994372674692, -17.50000000000002487 ) ) ;
#13415=ORIENTED_EDGE ( 'NONE', *, *, #5650, .T. ) ;
#13421=DIRECTION ( 'NONE',  ( 0.000000000000000000, 0.000000000000000000, -1.000000000000000000 ) ) ;
#13422=DIRECTION ( 'NONE',  ( 1.000000000000000000, 0.000000000000000000, 0.000000000000000000 ) ) ;
#13424=ADVANCED_FACE ( 'NONE', ( #14723 ), #12450, .F. ) ;
#13428=EDGE_LOOP ( 'NONE', ( #11492, #12961, #3012, #864 ) ) ;
#13429=CIRCLE ( 'NONE', #4612, 3.525000000000000355 ) ;
#13432=CARTESIAN_POINT ( 'NONE',  ( -70.00000000000000000, 17.53993994372673981, -13.99999999999999289 ) ) ;
#13437=CARTESIAN_POINT ( 'NONE',  ( -63.50000000000002842, 19.53993994372674692, -17.50000000000002487 ) ) ;
#13443=STYLED_ITEM ( 'NONE', ( #5996 ), #5544 ) ;
#13444=EDGE_CURVE ( 'NONE', #13055, #1161, #6295, .T. ) ;
#13456=ORIENTED_EDGE ( 'NONE', *, *, #9209, .F. ) ;
#13457=VERTEX_POINT ( 'NONE', #7415 ) ;
#13458=CARTESIAN_POINT ( 'NONE',  ( 164.0000000000000568, 64.53993994372673626, 13.29999999999999538 ) ) ;
#13462=EDGE_CURVE ( 'NONE', #14374, #10437, #9932, .T. ) ;
#13473=ORIENTED_EDGE ( 'NONE', *, *, #13724, .T. ) ;
#13474=CARTESIAN_POINT ( 'NONE',  ( 194.0000000000000568, 64.53993994372673626, 20.00000000000000355 ) ) ;
#13477=CARTESIAN_POINT ( 'NONE',  ( -35.99999999999995026, 64.53993994372673626, 15.00000000000139977 ) ) ;
#13478=DIRECTION ( 'NONE',  ( 0.000000000000000000, 0.000000000000000000, 1.000000000000000000 ) ) ;
#13481=AXIS2_PLACEMENT_3D ( 'NONE', #5093, #6207, #10067 ) ;
#13487=VERTEX_POINT ( 'NONE', #7482 ) ;
#13491=ORIENTED_EDGE ( 'NONE', *, *, #7204, .T. ) ;
#13493=LINE ( 'NONE', #14753, #4729 ) ;
#13500=DIRECTION ( 'NONE',  ( 3.965082230804130220E-16, -1.486905836551548832E-16, 1.000000000000000000 ) ) ;
#13512=DIRECTION ( 'NONE',  ( 0.000000000000000000, 0.000000000000000000, 1.000000000000000000 ) ) ;
#13513=DIRECTION ( 'NONE',  ( 0.000000000000000000, 0.000000000000000000, 1.000000000000000000 ) ) ;
#13514=VECTOR ( 'NONE', #13548, 1000.000000000000000 ) ;
#13516=AXIS2_PLACEMENT_3D ( 'NONE', #4293, #1924, #733 ) ;
#13528=ORIENTED_EDGE ( 'NONE', *, *, #5615, .T. ) ;
#13531=DIRECTION ( 'NONE',  ( 0.000000000000000000, -1.000000000000000000, -1.156482317317871478E-16 ) ) ;
#13532=CARTESIAN_POINT ( 'NONE',  ( 164.0000000000000568, 64.51493994372674479, 18.50000000000000711 ) ) ;
#13533=FACE_OUTER_BOUND ( 'NONE', #2751, .T. ) ;
#13534=DIRECTION ( 'NONE',  ( 0.000000000000000000, 0.000000000000000000, -1.000000000000000000 ) ) ;
#13537=DIRECTION ( 'NONE',  ( 1.000000000000000000, 0.000000000000000000, 0.000000000000000000 ) ) ;
#13538=FACE_OUTER_BOUND ( 'NONE', #12401, .T. ) ;
#13539=ORIENTED_EDGE ( 'NONE', *, *, #9571, .T. ) ;
#13548=DIRECTION ( 'NONE',  ( 3.965082230804130220E-16, 1.486905836551548832E-16, -1.000000000000000000 ) ) ;
#13549=EDGE_CURVE ( 'NONE', #7275, #4775, #12434, .T. ) ;
#13557=AXIS2_PLACEMENT_3D ( 'NONE', #10241, #13866, #3129 ) ;
#13560=ORIENTED_EDGE ( 'NONE', *, *, #5843, .F. ) ;
#13563=CARTESIAN_POINT ( 'NONE',  ( -35.99999999999995026, 64.51493994372674479, 11.50000000000139622 ) ) ;
#13566=EDGE_LOOP ( 'NONE', ( #15532, #11321, #3312, #8008, #6302, #11771 ) ) ;
#13568=EDGE_CURVE ( 'NONE', #8250, #10019, #9681, .T. ) ;
#13570=CARTESIAN_POINT ( 'NONE',  ( 64.00000000000005684, 64.53993994372673626, 15.00000000000070166 ) ) ;
#13580=ORIENTED_EDGE ( 'NONE', *, *, #5650, .F. ) ;
#13583=ADVANCED_FACE ( 'NONE', ( #1946 ), #4162, .F. ) ;
#13585=ORIENTED_EDGE ( 'NONE', *, *, #4797, .T. ) ;
#13590=MECHANICAL_DESIGN_GEOMETRIC_PRESENTATION_REPRESENTATION('',(#3030),#222);
#13592=CARTESIAN_POINT ( 'NONE',  ( 190.5000000000000568, 17.53993994372674692, -17.50000000000002487 ) ) ;
#13593=AXIS2_PLACEMENT_3D ( 'NONE', #2638, #2714, #13512 ) ;
#13596=ADVANCED_FACE ( 'NONE', ( #6642 ), #10180, .F. ) ;
#13597=CIRCLE ( 'NONE', #6820, 1.699999999999994849 ) ;
#13600=CONICAL_SURFACE ( 'NONE', #11865, 3.525000000000002132, 0.7853981633974482790 ) ;
#13617=CARTESIAN_POINT ( 'NONE',  ( -35.99999999999995026, 64.53993994372673626, 16.70000000000140261 ) ) ;
#13619=CARTESIAN_POINT ( 'NONE',  ( 215.1062858801516882, 25.86394065090268057, 18.00000000000000355 ) ) ;
#13621=CARTESIAN_POINT ( 'NONE',  ( 177.5000000000000853, 17.53993994372673271, 52.49999999999997868 ) ) ;
#13622=VERTEX_POINT ( 'NONE', #11597 ) ;
#13631=CARTESIAN_POINT ( 'NONE',  ( 14.00000000000004086, 64.53993994372673626, 11.47500000000104947 ) ) ;
#13632=DIRECTION ( 'NONE',  ( 0.000000000000000000, -1.000000000000000000, 0.000000000000000000 ) ) ;
#13637=ADVANCED_FACE ( 'NONE', ( #605 ), #4403, .F. ) ;
#13640=ORIENTED_EDGE ( 'NONE', *, *, #1445, .T. ) ;
#13649=AXIS2_PLACEMENT_3D ( 'NONE', #4904, #5131, #1569 ) ;
#13655=ORIENTED_EDGE ( 'NONE', *, *, #12744, .F. ) ;
#13657=EDGE_CURVE ( 'NONE', #13622, #9401, #15209, .T. ) ;
#13658=DIRECTION ( 'NONE',  ( -0.000000000000000000, 1.000000000000000000, -0.000000000000000000 ) ) ;
#13659=EDGE_CURVE ( 'NONE', #13457, #11511, #15047, .T. ) ;
#13665=ORIENTED_EDGE ( 'NONE', *, *, #9119, .T. ) ;
#13674=AXIS2_PLACEMENT_3D ( 'NONE', #9572, #14373, #3570 ) ;
#13677=CIRCLE ( 'NONE', #1359, 3.499999999999999556 ) ;
#13683=CARTESIAN_POINT ( 'NONE',  ( -35.99999999999995026, 64.53993994372673626, 13.30000000000139870 ) ) ;
#13687=VECTOR ( 'NONE', #10333, 1000.000000000000000 ) ;
#13693=DIRECTION ( 'NONE',  ( 0.000000000000000000, 0.000000000000000000, -1.000000000000000000 ) ) ;
#13695=VECTOR ( 'NONE', #10256, 1000.000000000000000 ) ;
#13696=DIRECTION ( 'NONE',  ( 0.000000000000000000, -1.000000000000000000, -1.156482317317871478E-16 ) ) ;
#13698=CARTESIAN_POINT ( 'NONE',  ( 194.0000000000000568, 59.53993994372674337, 10.00000000000000178 ) ) ;
#13699=AXIS2_PLACEMENT_3D ( 'NONE', #263, #340, #11187 ) ;
#13702=DIRECTION ( 'NONE',  ( -0.000000000000000000, 1.000000000000000000, -0.000000000000000000 ) ) ;
#13707=ORIENTED_EDGE ( 'NONE', *, *, #855, .T. ) ;
#13709=DIRECTION ( 'NONE',  ( 0.000000000000000000, -1.000000000000000000, 0.000000000000000000 ) ) ;
#13711=AXIS2_PLACEMENT_3D ( 'NONE', #12402, #8708, #1586 ) ;
#13713=( NAMED_UNIT ( * ) PLANE_ANGLE_UNIT ( ) SI_UNIT ( $, .RADIAN. ) );
#13718=DIRECTION ( 'NONE',  ( 0.000000000000000000, 0.000000000000000000, 1.000000000000000000 ) ) ;
#13724=EDGE_CURVE ( 'NONE', #9501, #14894, #10447, .T. ) ;
#13731=LINE ( 'NONE', #5141, #12871 ) ;
#13746=DIRECTION ( 'NONE',  ( 0.000000000000000000, 0.000000000000000000, 1.000000000000000000 ) ) ;
#13758=CIRCLE ( 'NONE', #1389, 3.500000000000003109 ) ;
#13759=FACE_OUTER_BOUND ( 'NONE', #13810, .T. ) ;
#13760=ORIENTED_EDGE ( 'NONE', *, *, #14370, .T. ) ;
#13769=AXIS2_PLACEMENT_3D ( 'NONE', #5480, #15240, #15085 ) ;
#13774=DIRECTION ( 'NONE',  ( 0.000000000000000000, 8.673617379884035472E-17, -1.000000000000000000 ) ) ;
#13780=DIRECTION ( 'NONE',  ( 0.000000000000000000, 0.000000000000000000, 1.000000000000000000 ) ) ;
#13782=ORIENTED_EDGE ( 'NONE', *, *, #8481, .T. ) ;
#13785=EDGE_LOOP ( 'NONE', ( #7143, #2468 ) ) ;
#13787=CARTESIAN_POINT ( 'NONE',  ( -63.50000000000002842, 17.53993994372674692, -17.50000000000002487 ) ) ;
#13806=DIRECTION ( 'NONE',  ( -0.000000000000000000, 1.000000000000000000, 1.156482317317871725E-16 ) ) ;
#13808=AXIS2_PLACEMENT_3D ( 'NONE', #2106, #11349, #4231 ) ;
#13810=EDGE_LOOP ( 'NONE', ( #3396, #13283, #9920, #1430, #13415, #3811, #14761, #14764 ) ) ;
#13817=CARTESIAN_POINT ( 'NONE',  ( 64.00000000000005684, 64.53993994372673626, 18.52500000000070202 ) ) ;
#13820=DIRECTION ( 'NONE',  ( 0.000000000000000000, -1.000000000000000000, 0.000000000000000000 ) ) ;
#13821=ORIENTED_EDGE ( 'NONE', *, *, #6433, .T. ) ;
#13836=CIRCLE ( 'NONE', #7541, 3.500000000000003109 ) ;
#13838=CARTESIAN_POINT ( 'NONE',  ( -63.50000000000002842, 17.53993994372674692, -17.50000000000002487 ) ) ;
#13841=EDGE_CURVE ( 'NONE', #5504, #6805, #5745, .T. ) ;
#13847=ORIENTED_EDGE ( 'NONE', *, *, #14251, .F. ) ;
#13857=AXIS2_PLACEMENT_3D ( 'NONE', #6317, #13478, #1400 ) ;
#13861=DIRECTION ( 'NONE',  ( 0.000000000000000000, 8.673617379884035472E-17, -1.000000000000000000 ) ) ;
#13866=DIRECTION ( 'NONE',  ( -0.000000000000000000, 1.000000000000000000, -0.000000000000000000 ) ) ;
#13867=LINE ( 'NONE', #13621, #10852 ) ;
#13890=CARTESIAN_POINT ( 'NONE',  ( 64.00000000000005684, 64.53993994372673626, 16.70000000000069207 ) ) ;
#13894=AXIS2_PLACEMENT_3D ( 'NONE', #7213, #12952, #9649 ) ;
#13902=LINE ( 'NONE', #8372, #4731 ) ;
#13904=CARTESIAN_POINT ( 'NONE',  ( 164.0000000000000568, 62.13993994372673768, 15.00000000000000355 ) ) ;
#13906=DIRECTION ( 'NONE',  ( -0.000000000000000000, 1.000000000000000000, -0.000000000000000000 ) ) ;
#13909=AXIS2_PLACEMENT_3D ( 'NONE', #13154, #2354, #4478 ) ;
#13910=CARTESIAN_POINT ( 'NONE',  ( 190.5000000000000568, 19.53993994372674692, -17.50000000000002487 ) ) ;
#13912=VERTEX_POINT ( 'NONE', #12475 ) ;
#13913=CARTESIAN_POINT ( 'NONE',  ( 64.00000000000005684, 62.13993994372673768, 16.70000000000069207 ) ) ;
#13916=DIRECTION ( 'NONE',  ( -0.000000000000000000, 1.000000000000000000, -0.000000000000000000 ) ) ;
#13930=ORIENTED_EDGE ( 'NONE', *, *, #10623, .F. ) ;
#13932=CIRCLE ( 'NONE', #10662, 3.500000000000001332 ) ;
#13934=DIRECTION ( 'NONE',  ( -0.000000000000000000, 1.000000000000000000, -0.000000000000000000 ) ) ;
#13938=DIRECTION ( 'NONE',  ( 8.659560562354932858E-17, 0.7071067811865474617, -0.7071067811865474617 ) ) ;
#13940=DIRECTION ( 'NONE',  ( 0.000000000000000000, 1.000000000000000000, 8.673617379884035472E-17 ) ) ;
#13942=CYLINDRICAL_SURFACE ( 'NONE', #13557, 1.699999999999994849 ) ;
#13947=AXIS2_PLACEMENT_3D ( 'NONE', #670, #2755, #1640 ) ;
#13951=LINE ( 'NONE', #6708, #11051 ) ;
#13960=VECTOR ( 'NONE', #7739, 1000.000000000000000 ) ;
#13961=DIRECTION ( 'NONE',  ( 0.000000000000000000, 0.000000000000000000, 1.000000000000000000 ) ) ;
#13970=VECTOR ( 'NONE', #6455, 1000.000000000000000 ) ;
#13971=DIRECTION ( 'NONE',  ( 0.000000000000000000, 0.000000000000000000, -1.000000000000000000 ) ) ;
#13975=ORIENTED_EDGE ( 'NONE', *, *, #6277, .T. ) ;
#13981=DIRECTION ( 'NONE',  ( 0.000000000000000000, 0.000000000000000000, 1.000000000000000000 ) ) ;
#13993=CYLINDRICAL_SURFACE ( 'NONE', #8340, 1.499999999999994449 ) ;
#13994=LINE ( 'NONE', #3182, #1500 ) ;
#14000=EDGE_CURVE ( 'NONE', #11935, #10092, #12634, .T. ) ;
#14020=EDGE_LOOP ( 'NONE', ( #5414, #14219, #10854, #9222 ) ) ;
#14021=DIRECTION ( 'NONE',  ( 0.000000000000000000, 0.000000000000000000, 1.000000000000000000 ) ) ;
#14032=LINE ( 'NONE', #6871, #6067 ) ;
#14035=( NAMED_UNIT ( * ) PLANE_ANGLE_UNIT ( ) SI_UNIT ( $, .RADIAN. ) );
#14040=CARTESIAN_POINT ( 'NONE',  ( -110.0000000000000426, 19.53993994372674337, 9.999999999999998224 ) ) ;
#14044=ORIENTED_EDGE ( 'NONE', *, *, #8531, .T. ) ;
#14050=EDGE_CURVE ( 'NONE', #14894, #10019, #13902, .T. ) ;
#14051=ADVANCED_FACE ( 'NONE', ( #3615 ), #1953, .F. ) ;
#14056=FACE_BOUND ( 'NONE', #10115, .T. ) ;
#14058=VECTOR ( 'NONE', #669, 1000.000000000000000 ) ;
#14071=CONICAL_SURFACE ( 'NONE', #5754, 3.525000000000000355, 0.7853981633975176679 ) ;
#14073=CARTESIAN_POINT ( 'NONE',  ( 184.0000000000000568, 17.53993994372673981, -13.99999999999999289 ) ) ;
#14082=ORIENTED_EDGE ( 'NONE', *, *, #9905, .F. ) ;
#14085=EDGE_LOOP ( 'NONE', ( #3888, #3294, #3291, #2058 ) ) ;
#14090=CARTESIAN_POINT ( 'NONE',  ( 164.0000000000000568, 64.53993994372673626, 15.00000000000000355 ) ) ;
#14092=LINE ( 'NONE', #11668, #6845 ) ;
#14093=CIRCLE ( 'NONE', #464, 1.699999999999993072 ) ;
#14094=ORIENTED_EDGE ( 'NONE', *, *, #917, .F. ) ;
#14095=VERTEX_POINT ( 'NONE', #13231 ) ;
#14097=CARTESIAN_POINT ( 'NONE',  ( 164.0000000000000568, 59.53993994372674337, 16.70000000000000995 ) ) ;
#14106=LINE ( 'NONE', #9164, #5668 ) ;
#14111=EDGE_CURVE ( 'NONE', #8731, #899, #1443, .T. ) ;
#14112=VECTOR ( 'NONE', #11476, 1000.000000000000000 ) ;
#14115=ORIENTED_EDGE ( 'NONE', *, *, #2051, .T. ) ;
#14117=CARTESIAN_POINT ( 'NONE',  ( 64.00000000000005684, 62.13993994372673768, 15.00000000000070166 ) ) ;
#14121=VECTOR ( 'NONE', #6181, 1000.000000000000000 ) ;
#14137=DIRECTION ( 'NONE',  ( 0.000000000000000000, -1.000000000000000000, 0.000000000000000000 ) ) ;
#14141=DIRECTION ( 'NONE',  ( 0.000000000000000000, 0.000000000000000000, 1.000000000000000000 ) ) ;
#14148=VECTOR ( 'NONE', #23, 1000.000000000000000 ) ;
#14150=LINE ( 'NONE', #6026, #5689 ) ;
#14152=CARTESIAN_POINT ( 'NONE',  ( -110.0000000000000426, 59.53993994372674337, 25.00000000000000000 ) ) ;
#14156=EDGE_LOOP ( 'NONE', ( #9554, #2727 ) ) ;
#14162=CARTESIAN_POINT ( 'NONE',  ( 14.00000000000004086, 59.53993994372674337, 16.70000000000105089 ) ) ;
#14164=EDGE_LOOP ( 'NONE', ( #10527, #7446, #14733, #3273 ) ) ;
#14175=EDGE_CURVE ( 'NONE', #411, #6899, #4480, .T. ) ;
#14176=DIRECTION ( 'NONE',  ( -0.000000000000000000, -1.000000000000000000, -0.000000000000000000 ) ) ;
#14181=FACE_OUTER_BOUND ( 'NONE', #14020, .T. ) ;
#14185=DIRECTION ( 'NONE',  ( -0.000000000000000000, 1.000000000000000000, -0.000000000000000000 ) ) ;
#14189=ORIENTED_EDGE ( 'NONE', *, *, #5457, .T. ) ;
#14192=DIRECTION ( 'NONE',  ( 0.000000000000000000, 0.000000000000000000, 1.000000000000000000 ) ) ;
#14193=CIRCLE ( 'NONE', #7413, 2.000000000000000000 ) ;
#14196=DIRECTION ( 'NONE',  ( -0.000000000000000000, 1.000000000000000000, -0.000000000000000000 ) ) ;
#14201=AXIS2_PLACEMENT_3D ( 'NONE', #15437, #13227, #14489 ) ;
#14205=FACE_OUTER_BOUND ( 'NONE', #3638, .T. ) ;
#14208=ORIENTED_EDGE ( 'NONE', *, *, #13117, .F. ) ;
#14219=ORIENTED_EDGE ( 'NONE', *, *, #10958, .F. ) ;
#14221=ORIENTED_EDGE ( 'NONE', *, *, #13234, .T. ) ;
#14222=ADVANCED_FACE ( 'NONE', ( #8824 ), #3991, .F. ) ;
#14235=FACE_BOUND ( 'NONE', #2610, .T. ) ;
#14236=EDGE_CURVE ( 'NONE', #11227, #9977, #5003, .T. ) ;
#14237=DIRECTION ( 'NONE',  ( 0.000000000000000000, 0.000000000000000000, 1.000000000000000000 ) ) ;
#14249=EDGE_CURVE ( 'NONE', #14286, #15409, #4746, .T. ) ;
#14251=EDGE_CURVE ( 'NONE', #6589, #2137, #10892, .T. ) ;
#14266=CARTESIAN_POINT ( 'NONE',  ( 64.00000000000005684, 62.13993994372673768, 13.30000000000070948 ) ) ;
#14281=CIRCLE ( 'NONE', #10520, 1.699999999999993072 ) ;
#14283=DIRECTION ( 'NONE',  ( -0.000000000000000000, 1.000000000000000000, -0.000000000000000000 ) ) ;
#14286=VERTEX_POINT ( 'NONE', #3688 ) ;
#14289=VERTEX_POINT ( 'NONE', #8519 ) ;
#14302=AXIS2_PLACEMENT_3D ( 'NONE', #11910, #10808, #7923 ) ;
#14306=EDGE_CURVE ( 'NONE', #12693, #4660, #3923, .T. ) ;
#14311=VECTOR ( 'NONE', #9775, 1000.000000000000114 ) ;
#14312=EDGE_CURVE ( 'NONE', #591, #2912, #14653, .T. ) ;
#14316=FACE_OUTER_BOUND ( 'NONE', #1182, .T. ) ;
#14320=DIRECTION ( 'NONE',  ( 0.000000000000000000, 1.000000000000000000, 8.673617379884035472E-17 ) ) ;
#14332=EDGE_CURVE ( 'NONE', #13487, #14978, #953, .T. ) ;
#14334=EDGE_CURVE ( 'NONE', #5937, #9838, #2988, .T. ) ;
#14335=DIRECTION ( 'NONE',  ( -0.000000000000000000, -0.000000000000000000, 1.000000000000000000 ) ) ;
#14336=AXIS2_PLACEMENT_3D ( 'NONE', #5927, #9565, #7212 ) ;
#14355=VECTOR ( 'NONE', #6106, 1000.000000000000000 ) ;
#14356=ORIENTED_EDGE ( 'NONE', *, *, #3700, .T. ) ;
#14359=CARTESIAN_POINT ( 'NONE',  ( -85.99999999999994316, 59.53993994372674337, 13.30000000000175575 ) ) ;
#14367=LINE ( 'NONE', #11937, #7876 ) ;
#14370=EDGE_CURVE ( 'NONE', #13055, #14289, #6541, .T. ) ;
#14373=DIRECTION ( 'NONE',  ( -0.000000000000000000, 1.000000000000000000, -0.000000000000000000 ) ) ;
#14374=VERTEX_POINT ( 'NONE', #11342 ) ;
#14382=ORIENTED_EDGE ( 'NONE', *, *, #9029, .F. ) ;
#14386=ORIENTED_EDGE ( 'NONE', *, *, #2719, .T. ) ;
#14387=DIRECTION ( 'NONE',  ( -0.000000000000000000, 1.000000000000000000, -0.000000000000000000 ) ) ;
#14389=LINE ( 'NONE', #3660, #9831 ) ;
#14393=ADVANCED_FACE ( 'NONE', ( #662 ), #12669, .F. ) ;
#14398=CYLINDRICAL_SURFACE ( 'NONE', #14491, 3.500000000000004885 ) ;
#14400=CYLINDRICAL_SURFACE ( 'NONE', #4756, 3.500000000000003109 ) ;
#14404=CARTESIAN_POINT ( 'NONE',  ( 14.00000000000004086, 64.53993994372673626, 18.52500000000105018 ) ) ;
#14405=EDGE_LOOP ( 'NONE', ( #14382, #3502, #10481, #9005 ) ) ;
#14412=DIRECTION ( 'NONE',  ( -1.000000000000000000, 0.000000000000000000, 0.000000000000000000 ) ) ;
#14422=DIRECTION ( 'NONE',  ( -1.000000000000000000, 0.000000000000000000, 0.000000000000000000 ) ) ;
#14426=DIRECTION ( 'NONE',  ( 0.000000000000000000, 0.000000000000000000, 1.000000000000000000 ) ) ;
#14431=CYLINDRICAL_SURFACE ( 'NONE', #13343, 1.699999999999996625 ) ;
#14433=ADVANCED_FACE ( 'NONE', ( #5342 ), #13942, .F. ) ;
#14445=EDGE_LOOP ( 'NONE', ( #6492, #27 ) ) ;
#14450=ORIENTED_EDGE ( 'NONE', *, *, #1796, .T. ) ;
#14458=LINE ( 'NONE', #9821, #10838 ) ;
#14464=AXIS2_PLACEMENT_3D ( 'NONE', #7989, #9321, #15291 ) ;
#14467=DIRECTION ( 'NONE',  ( 0.000000000000000000, 0.000000000000000000, 1.000000000000000000 ) ) ;
#14468=EDGE_LOOP ( 'NONE', ( #14588, #694, #9675, #6009 ) ) ;
#14479=CARTESIAN_POINT ( 'NONE',  ( 184.0000000000000568, 17.53993994372673981, -13.99999999999999289 ) ) ;
#14485=DIRECTION ( 'NONE',  ( -0.000000000000000000, 1.000000000000000000, -0.000000000000000000 ) ) ;
#14489=DIRECTION ( 'NONE',  ( 0.000000000000000000, 0.000000000000000000, 1.000000000000000000 ) ) ;
#14491=AXIS2_PLACEMENT_3D ( 'NONE', #8202, #15571, #11970 ) ;
#14492=ADVANCED_FACE ( 'NONE', ( #6622 ), #14071, .F. ) ;
#14494=DIRECTION ( 'NONE',  ( -0.000000000000000000, 1.000000000000000000, 1.156482317317871725E-16 ) ) ;
#14498=ORIENTED_EDGE ( 'NONE', *, *, #11111, .T. ) ;
#14503=CARTESIAN_POINT ( 'NONE',  ( -110.0000000000000426, 19.53993994372674337, 24.99999999999999645 ) ) ;
#14504=CARTESIAN_POINT ( 'NONE',  ( 64.00000000000005684, 64.53993994372673626, 11.50000000000069811 ) ) ;
#14521=CIRCLE ( 'NONE', #2695, 3.500000000000004885 ) ;
#14525=DIRECTION ( 'NONE',  ( 0.000000000000000000, -1.000000000000000000, 0.000000000000000000 ) ) ;
#14528=ADVANCED_FACE ( 'NONE', ( #4385 ), #9216, .F. ) ;
#14532=DIRECTION ( 'NONE',  ( -0.000000000000000000, 1.000000000000000000, -0.000000000000000000 ) ) ;
#14535=ORIENTED_EDGE ( 'NONE', *, *, #4994, .T. ) ;
#14540=FACE_OUTER_BOUND ( 'NONE', #6499, .T. ) ;
#14541=DIRECTION ( 'NONE',  ( -0.000000000000000000, 1.000000000000000000, -0.000000000000000000 ) ) ;
#14548=AXIS2_PLACEMENT_3D ( 'NONE', #9468, #4639, #15596 ) ;
#14569=DIRECTION ( 'NONE',  ( -0.000000000000000000, 1.000000000000000000, -0.000000000000000000 ) ) ;
#14572=DIRECTION ( 'NONE',  ( 0.000000000000000000, 0.000000000000000000, 1.000000000000000000 ) ) ;
#14581=DIRECTION ( 'NONE',  ( 0.000000000000000000, -1.000000000000000000, 0.000000000000000000 ) ) ;
#14582=CARTESIAN_POINT ( 'NONE',  ( 64.00000000000005684, 56.53993994372675047, 15.00000000000070166 ) ) ;
#14588=ORIENTED_EDGE ( 'NONE', *, *, #8034, .F. ) ;
#14592=VECTOR ( 'NONE', #11653, 1000.000000000000000 ) ;
#14595=ORIENTED_EDGE ( 'NONE', *, *, #5457, .F. ) ;
#14599=ORIENTED_EDGE ( 'NONE', *, *, #8760, .F. ) ;
#14601=CARTESIAN_POINT ( 'NONE',  ( -110.0000000000000426, 19.53993994372674337, 24.99999999999999645 ) ) ;
#14602=ADVANCED_FACE ( 'NONE', ( #11972, #12910, #5890 ), #5734, .F. ) ;
#14609=EDGE_LOOP ( 'NONE', ( #6201, #13782, #15401, #5000 ) ) ;
#14610=PLANE ( 'NONE',  #11712 ) ;
#14612=EDGE_LOOP ( 'NONE', ( #2966, #5941 ) ) ;
#14620=AXIS2_PLACEMENT_3D ( 'NONE', #794, #2875, #10137 ) ;
#14626=EDGE_CURVE ( 'NONE', #3946, #10635, #7004, .T. ) ;
#14643=ORIENTED_EDGE ( 'NONE', *, *, #3662, .F. ) ;
#14650=AXIS2_PLACEMENT_3D ( 'NONE', #5860, #9566, #2299 ) ;
#14653=LINE ( 'NONE', #4960, #14311 ) ;
#14655=DIRECTION ( 'NONE',  ( 0.000000000000000000, 0.000000000000000000, 1.000000000000000000 ) ) ;
#14656=ORIENTED_EDGE ( 'NONE', *, *, #346, .T. ) ;
#14657=DIRECTION ( 'NONE',  ( 0.000000000000000000, -1.000000000000000000, -1.156482317317871478E-16 ) ) ;
#14693=EDGE_LOOP ( 'NONE', ( #13379, #10263 ) ) ;
#14709=FACE_OUTER_BOUND ( 'NONE', #3672, .T. ) ;
#14710=ADVANCED_FACE ( 'NONE', ( #4780 ), #14400, .F. ) ;
#14715=AXIS2_PLACEMENT_3D ( 'NONE', #8738, #13531, #12355 ) ;
#14716=EDGE_LOOP ( 'NONE', ( #7230, #5737, #7224, #7843, #14961 ) ) ;
#14717=ORIENTED_EDGE ( 'NONE', *, *, #2642, .F. ) ;
#14722=AXIS2_PLACEMENT_3D ( 'NONE', #9701, #15515, #11988 ) ;
#14723=FACE_OUTER_BOUND ( 'NONE', #6750, .T. ) ;
#14724=DIRECTION ( 'NONE',  ( 0.000000000000000000, 1.000000000000000000, 0.000000000000000000 ) ) ;
#14733=ORIENTED_EDGE ( 'NONE', *, *, #1006, .T. ) ;
#14753=CARTESIAN_POINT ( 'NONE',  ( -85.99999999999994316, 64.53993994372673626, 11.47500000000174758 ) ) ;
#14758=VERTEX_POINT ( 'NONE', #7401 ) ;
#14761=ORIENTED_EDGE ( 'NONE', *, *, #11252, .T. ) ;
#14764=ORIENTED_EDGE ( 'NONE', *, *, #244, .T. ) ;
#14770=CARTESIAN_POINT ( 'NONE',  ( -63.50000000000002842, 19.53993994372674692, -17.50000000000002487 ) ) ;
#14774=DIRECTION ( 'NONE',  ( -0.000000000000000000, 1.000000000000000000, -0.000000000000000000 ) ) ;
#14776=CARTESIAN_POINT ( 'NONE',  ( -108.0000000000000568, 64.53993994372673626, 10.00000000000000178 ) ) ;
#14777=DIRECTION ( 'NONE',  ( 0.000000000000000000, -1.156482317317871725E-16, 1.000000000000000000 ) ) ;
#14787=ORIENTED_EDGE ( 'NONE', *, *, #4302, .T. ) ;
#14789=CARTESIAN_POINT ( 'NONE',  ( 164.0000000000000568, 59.53993994372674337, 16.70000000000000995 ) ) ;
#14793=DIRECTION ( 'NONE',  ( -0.000000000000000000, 1.000000000000000000, 1.156482317317871725E-16 ) ) ;
#14794=CARTESIAN_POINT ( 'NONE',  ( 164.0000000000000568, 64.53993994372673626, 15.00000000000000355 ) ) ;
#14800=VECTOR ( 'NONE', #10483, 1000.000000000000000 ) ;
#14801=ORIENTED_EDGE ( 'NONE', *, *, #13841, .T. ) ;
#14807=LINE ( 'NONE', #2916, #13960 ) ;
#14815=VECTOR ( 'NONE', #5425, 1000.000000000000000 ) ;
#14824=ORIENTED_EDGE ( 'NONE', *, *, #7859, .T. ) ;
#14830=LINE ( 'NONE', #4027, #8164 ) ;
#14837=VERTEX_POINT ( 'NONE', #8434 ) ;
#14840=ADVANCED_FACE ( 'NONE', ( #14709 ), #8655, .F. ) ;
#14844=EDGE_LOOP ( 'NONE', ( #3004, #10473 ) ) ;
#14847=EDGE_CURVE ( 'NONE', #5951, #11227, #12266, .T. ) ;
#14862=LINE ( 'NONE', #13683, #1466 ) ;
#14872=VECTOR ( 'NONE', #13396, 1000.000000000000000 ) ;
#14877=LINE ( 'NONE', #13617, #3397 ) ;
#14884=DIRECTION ( 'NONE',  ( -1.000000000000000000, 0.000000000000000000, 0.000000000000000000 ) ) ;
#14891=DIRECTION ( 'NONE',  ( 0.000000000000000000, 0.000000000000000000, -1.000000000000000000 ) ) ;
#14894=VERTEX_POINT ( 'NONE', #1768 ) ;
#14900=DIRECTION ( 'NONE',  ( -0.000000000000000000, 1.000000000000000000, 1.156482317317871725E-16 ) ) ;
#14903=EDGE_CURVE ( 'NONE', #2217, #11305, #14862, .T. ) ;
#14908=VECTOR ( 'NONE', #13938, 1000.000000000000114 ) ;
#14917=AXIS2_PLACEMENT_3D ( 'NONE', #5164, #14777, #10942 ) ;
#14927=CARTESIAN_POINT ( 'NONE',  ( 114.0000000000000568, 62.13993994372673768, 15.00000000000035172 ) ) ;
#14929=CARTESIAN_POINT ( 'NONE',  ( -70.00000000000000000, 17.53993994372673981, -10.99999999999999822 ) ) ;
#14931=FACE_OUTER_BOUND ( 'NONE', #2527, .T. ) ;
#14933=DIRECTION ( 'NONE',  ( -1.000000000000000000, 0.000000000000000000, 0.000000000000000000 ) ) ;
#14938=ORIENTED_EDGE ( 'NONE', *, *, #8462, .T. ) ;
#14942=DIRECTION ( 'NONE',  ( -0.000000000000000000, 1.000000000000000000, -0.000000000000000000 ) ) ;
#14958=ORIENTED_EDGE ( 'NONE', *, *, #6901, .T. ) ;
#14960=ORIENTED_EDGE ( 'NONE', *, *, #13086, .T. ) ;
#14961=ORIENTED_EDGE ( 'NONE', *, *, #12915, .F. ) ;
#14965=CARTESIAN_POINT ( 'NONE',  ( 114.0000000000000568, 56.53993994372675047, 15.00000000000035172 ) ) ;
#14972=CARTESIAN_POINT ( 'NONE',  ( 184.0000000000000568, 17.53993994372673981, -12.49999999999999467 ) ) ;
#14973=CIRCLE ( 'NONE', #1122, 6.999999999999992006 ) ;
#14974=LINE ( 'NONE', #12301, #13403 ) ;
#14975=DIRECTION ( 'NONE',  ( 0.000000000000000000, -1.000000000000000000, 0.000000000000000000 ) ) ;
#14976=ORIENTED_EDGE ( 'NONE', *, *, #6650, .F. ) ;
#14978=VERTEX_POINT ( 'NONE', #11488 ) ;
#14980=LINE ( 'NONE', #13890, #11894 ) ;
#14994=EDGE_CURVE ( 'NONE', #2210, #591, #12729, .T. ) ;
#14998=AXIS2_PLACEMENT_3D ( 'NONE', #13904, #11623, #13981 ) ;
#15001=ORIENTED_EDGE ( 'NONE', *, *, #13360, .T. ) ;
#15011=AXIS2_PLACEMENT_3D ( 'NONE', #7125, #3143, #12761 ) ;
#15013=ADVANCED_FACE ( 'NONE', ( #3042 ), #6753, .F. ) ;
#15017=LINE ( 'NONE', #7869, #6704 ) ;
#15019=DIRECTION ( 'NONE',  ( -0.000000000000000000, 1.000000000000000000, -0.000000000000000000 ) ) ;
#15030=VERTEX_POINT ( 'NONE', #9427 ) ;
#15036=CARTESIAN_POINT ( 'NONE',  ( 224.0000000000000853, 22.53993994372673981, 24.99999999999999645 ) ) ;
#15038=EDGE_CURVE ( 'NONE', #8632, #15428, #14093, .T. ) ;
#15039=ORIENTED_EDGE ( 'NONE', *, *, #2911, .F. ) ;
#15042=CARTESIAN_POINT ( 'NONE',  ( -110.0000000000000426, 56.53993994372675047, 25.00000000000000000 ) ) ;
#15047=LINE ( 'NONE', #2994, #15213 ) ;
#15057=CARTESIAN_POINT ( 'NONE',  ( 177.5000000000000853, 19.53993994372674692, -17.50000000000002487 ) ) ;
#15058=EDGE_LOOP ( 'NONE', ( #6409, #7053 ) ) ;
#15063=CARTESIAN_POINT ( 'NONE',  ( 184.0000000000000568, 19.53993994372674337, -13.99999999999999289 ) ) ;
#15076=DIRECTION ( 'NONE',  ( 0.000000000000000000, -1.000000000000000000, 0.000000000000000000 ) ) ;
#15081=ORIENTED_EDGE ( 'NONE', *, *, #747, .T. ) ;
#15085=DIRECTION ( 'NONE',  ( 0.000000000000000000, 0.000000000000000000, 1.000000000000000000 ) ) ;
#15101=EDGE_CURVE ( 'NONE', #12980, #8626, #13118, .T. ) ;
#15105=DIRECTION ( 'NONE',  ( 0.000000000000000000, -1.000000000000000000, 0.000000000000000000 ) ) ;
#15107=DIRECTION ( 'NONE',  ( 0.000000000000000000, 0.000000000000000000, 1.000000000000000000 ) ) ;
#15108=ORIENTED_EDGE ( 'NONE', *, *, #9556, .T. ) ;
#15109=AXIS2_PLACEMENT_3D ( 'NONE', #3033, #7864, #14933 ) ;
#15112=CARTESIAN_POINT ( 'NONE',  ( 164.0000000000000568, 64.53993994372673626, 15.00000000000000355 ) ) ;
#15113=CYLINDRICAL_SURFACE ( 'NONE', #7315, 1.499999999999997780 ) ;
#15122=CIRCLE ( 'NONE', #6833, 4.999999999999990230 ) ;
#15123=CARTESIAN_POINT ( 'NONE',  ( -76.50000000000002842, 19.53993994372674337, 24.99999999999999645 ) ) ;
#15127=CARTESIAN_POINT ( 'NONE',  ( 177.5000000000000853, 19.53993994372674692, -17.50000000000002487 ) ) ;
#15128=VECTOR ( 'NONE', #3743, 1000.000000000000000 ) ;
#15129=CARTESIAN_POINT ( 'NONE',  ( 224.0000000000000853, 22.53993994372673981, 13.00000000000000178 ) ) ;
#15130=AXIS2_PLACEMENT_3D ( 'NONE', #7380, #9820, #14572 ) ;
#15131=DIRECTION ( 'NONE',  ( 0.000000000000000000, 1.000000000000000000, 8.673617379884035472E-17 ) ) ;
#15139=LINE ( 'NONE', #14040, #5108 ) ;
#15140=CARTESIAN_POINT ( 'NONE',  ( 14.00000000000004086, 64.53993994372673626, 15.00000000000104983 ) ) ;
#15141=DIRECTION ( 'NONE',  ( 0.000000000000000000, 0.000000000000000000, 1.000000000000000000 ) ) ;
#15142=AXIS2_PLACEMENT_3D ( 'NONE', #14927, #4119, #13746 ) ;
#15143=AXIS2_PLACEMENT_3D ( 'NONE', #10097, #1714, #6394 ) ;
#15148=ORIENTED_EDGE ( 'NONE', *, *, #4517, .F. ) ;
#15150=VERTEX_POINT ( 'NONE', #3347 ) ;
#15156=AXIS2_PLACEMENT_3D ( 'NONE', #7828, #14900, #11368 ) ;
#15158=VERTEX_POINT ( 'NONE', #10378 ) ;
#15163=FACE_OUTER_BOUND ( 'NONE', #10497, .T. ) ;
#15166=EDGE_CURVE ( 'NONE', #9501, #8250, #15171, .T. ) ;
#15167=CARTESIAN_POINT ( 'NONE',  ( 164.0000000000000568, 64.53993994372673626, 11.47500000000000320 ) ) ;
#15171=LINE ( 'NONE', #14073, #9568 ) ;
#15176=VECTOR ( 'NONE', #12017, 1000.000000000000000 ) ;
#15191=EDGE_CURVE ( 'NONE', #1434, #15197, #9741, .T. ) ;
#15192=DIRECTION ( 'NONE',  ( -0.000000000000000000, 1.000000000000000000, 0.000000000000000000 ) ) ;
#15197=VERTEX_POINT ( 'NONE', #1277 ) ;
#15203=VECTOR ( 'NONE', #2607, 1000.000000000000000 ) ;
#15209=LINE ( 'NONE', #15129, #13695 ) ;
#15213=VECTOR ( 'NONE', #9163, 1000.000000000000000 ) ;
#15214=SHAPE_REPRESENTATION_RELATIONSHIP ( 'NONE' , 'NONE' ,  #3806, #6418 ) ;
#15222=DIRECTION ( 'NONE',  ( 0.000000000000000000, -1.000000000000000000, -1.486905836551548832E-16 ) ) ;
#15237=DIRECTION ( 'NONE',  ( -0.000000000000000000, 1.000000000000000000, -0.000000000000000000 ) ) ;
#15239=CARTESIAN_POINT ( 'NONE',  ( -110.0000000000000426, 59.53993994372674337, 25.00000000000000000 ) ) ;
#15240=DIRECTION ( 'NONE',  ( -0.000000000000000000, 1.000000000000000000, 1.156482317317871725E-16 ) ) ;
#15243=PLANE ( 'NONE',  #1242 ) ;
#15248=ORIENTED_EDGE ( 'NONE', *, *, #11565, .F. ) ;
#15251=ORIENTED_EDGE ( 'NONE', *, *, #9805, .F. ) ;
#15254=EDGE_CURVE ( 'NONE', #5209, #2490, #14458, .T. ) ;
#15265=ORIENTED_EDGE ( 'NONE', *, *, #12696, .F. ) ;
#15271=CARTESIAN_POINT ( 'NONE',  ( 64.00000000000005684, 59.53993994372674337, 15.00000000000070166 ) ) ;
#15281=DIRECTION ( 'NONE',  ( 0.000000000000000000, 8.673617379884035472E-17, -1.000000000000000000 ) ) ;
#15287=CARTESIAN_POINT ( 'NONE',  ( 164.0000000000000568, 64.53993994372673626, 18.52500000000000213 ) ) ;
#15291=DIRECTION ( 'NONE',  ( 0.000000000000000000, 1.000000000000000000, 0.000000000000000000 ) ) ;
#15312=DIRECTION ( 'NONE',  ( -0.000000000000000000, 1.000000000000000000, -0.000000000000000000 ) ) ;
#15313=AXIS2_PLACEMENT_3D ( 'NONE', #272, #2592, #186 ) ;
#15314=FACE_OUTER_BOUND ( 'NONE', #14164, .T. ) ;
#15317=FILL_AREA_STYLE ('',( #2149 ) ) ;
#15329=DIRECTION ( 'NONE',  ( 0.000000000000000000, 0.000000000000000000, 1.000000000000000000 ) ) ;
#15342=CARTESIAN_POINT ( 'NONE',  ( -85.99999999999994316, 64.53993994372673626, 15.00000000000174794 ) ) ;
#15350=DIRECTION ( 'NONE',  ( -0.000000000000000000, 1.000000000000000000, -0.000000000000000000 ) ) ;
#15354=VECTOR ( 'NONE', #198, 1000.000000000000000 ) ;
#15370=CARTESIAN_POINT ( 'NONE',  ( -85.99999999999994316, 56.53993994372675047, 13.30000000000175575 ) ) ;
#15371=ORIENTED_EDGE ( 'NONE', *, *, #7094, .T. ) ;
#15372=DIRECTION ( 'NONE',  ( -0.000000000000000000, 1.000000000000000000, -0.000000000000000000 ) ) ;
#15375=EDGE_CURVE ( 'NONE', #4912, #2296, #13335, .T. ) ;
#15379=ORIENTED_EDGE ( 'NONE', *, *, #12284, .F. ) ;
#15380=PRODUCT_DEFINITION ( 'UNKNOWN', '', #8307, #438 ) ;
#15391=CARTESIAN_POINT ( 'NONE',  ( 164.0000000000000568, 56.53993994372675047, 15.00000000000000355 ) ) ;
#15401=ORIENTED_EDGE ( 'NONE', *, *, #4891, .T. ) ;
#15409=VERTEX_POINT ( 'NONE', #12479 ) ;
#15412=FACE_BOUND ( 'NONE', #5884, .T. ) ;
#15413=VECTOR ( 'NONE', #5909, 1000.000000000000000 ) ;
#15415=EDGE_CURVE ( 'NONE', #2912, #12821, #5776, .T. ) ;
#15419=ORIENTED_EDGE ( 'NONE', *, *, #12224, .T. ) ;
#15420=CARTESIAN_POINT ( 'NONE',  ( 177.5000000000000853, 17.53993994372673271, 52.49999999999997868 ) ) ;
#15427=ORIENTED_EDGE ( 'NONE', *, *, #9080, .T. ) ;
#15428=VERTEX_POINT ( 'NONE', #12638 ) ;
#15437=CARTESIAN_POINT ( 'NONE',  ( 164.0000000000000568, 62.13993994372673768, 15.00000000000000355 ) ) ;
#15438=CARTESIAN_POINT ( 'NONE',  ( 14.00000000000004086, 64.53993994372673626, 13.30000000000105231 ) ) ;
#15439=CYLINDRICAL_SURFACE ( 'NONE', #1253, 1.700000000000001954 ) ;
#15447=DIRECTION ( 'NONE',  ( 0.000000000000000000, 0.000000000000000000, 1.000000000000000000 ) ) ;
#15456=ORIENTED_EDGE ( 'NONE', *, *, #14312, .F. ) ;
#15468=ADVANCED_FACE ( 'NONE', ( #7765 ), #12299, .F. ) ;
#15470=EDGE_LOOP ( 'NONE', ( #13209, #2037 ) ) ;
#15478=VERTEX_POINT ( 'NONE', #13017 ) ;
#15480=VECTOR ( 'NONE', #14724, 1000.000000000000000 ) ;
#15487=ADVANCED_FACE ( 'NONE', ( #11856 ), #4584, .F. ) ;
#15500=CARTESIAN_POINT ( 'NONE',  ( 0.000000000000000000, 17.53993994372673981, 2.674108611355829274E-15 ) ) ;
#15504=AXIS2_PLACEMENT_3D ( 'NONE', #7451, #14532, #8711 ) ;
#15514=DIRECTION ( 'NONE',  ( -0.000000000000000000, 0.000000000000000000, 1.000000000000000000 ) ) ;
#15515=DIRECTION ( 'NONE',  ( 0.000000000000000000, 1.000000000000000000, 0.000000000000000000 ) ) ;
#15526=DIRECTION ( 'NONE',  ( 0.000000000000000000, -0.000000000000000000, -1.000000000000000000 ) ) ;
#15527=DIRECTION ( 'NONE',  ( 0.000000000000000000, 0.000000000000000000, -1.000000000000000000 ) ) ;
#15528=ORIENTED_EDGE ( 'NONE', *, *, #8741, .T. ) ;
#15532=ORIENTED_EDGE ( 'NONE', *, *, #3820, .T. ) ;
#15535=EDGE_LOOP ( 'NONE', ( #5015, #10033, #7063, #848 ) ) ;
#15547=( LENGTH_UNIT ( ) NAMED_UNIT ( * ) SI_UNIT ( .MILLI., .METRE. ) );
#15571=DIRECTION ( 'NONE',  ( -0.000000000000000000, 1.000000000000000000, -0.000000000000000000 ) ) ;
#15579=FACE_OUTER_BOUND ( 'NONE', #4942, .T. ) ;
#15580=VECTOR ( 'NONE', #6096, 1000.000000000000000 ) ;
#15596=DIRECTION ( 'NONE',  ( 0.000000000000000000, 0.000000000000000000, 1.000000000000000000 ) ) ;
#15597=CARTESIAN_POINT ( 'NONE',  ( 184.0000000000000568, 17.53993994372673271, 48.99999999999997158 ) ) ;
#15598=ORIENTED_EDGE ( 'NONE', *, *, #11840, .T. ) ;
#15600=CARTESIAN_POINT ( 'NONE',  ( 200.1062858801516597, 40.86394065090267702, 18.00000000000000355 ) ) ;
#15601=DIRECTION ( 'NONE',  ( 0.000000000000000000, 0.7071067811865474617, 0.7071067811865474617 ) ) ;
#15608=CIRCLE ( 'NONE', #15109, 6.999999999999978684 ) ;
#15612=ORIENTED_EDGE ( 'NONE', *, *, #1988, .F. ) ;
ENDSEC;
END-ISO-10303-21;
